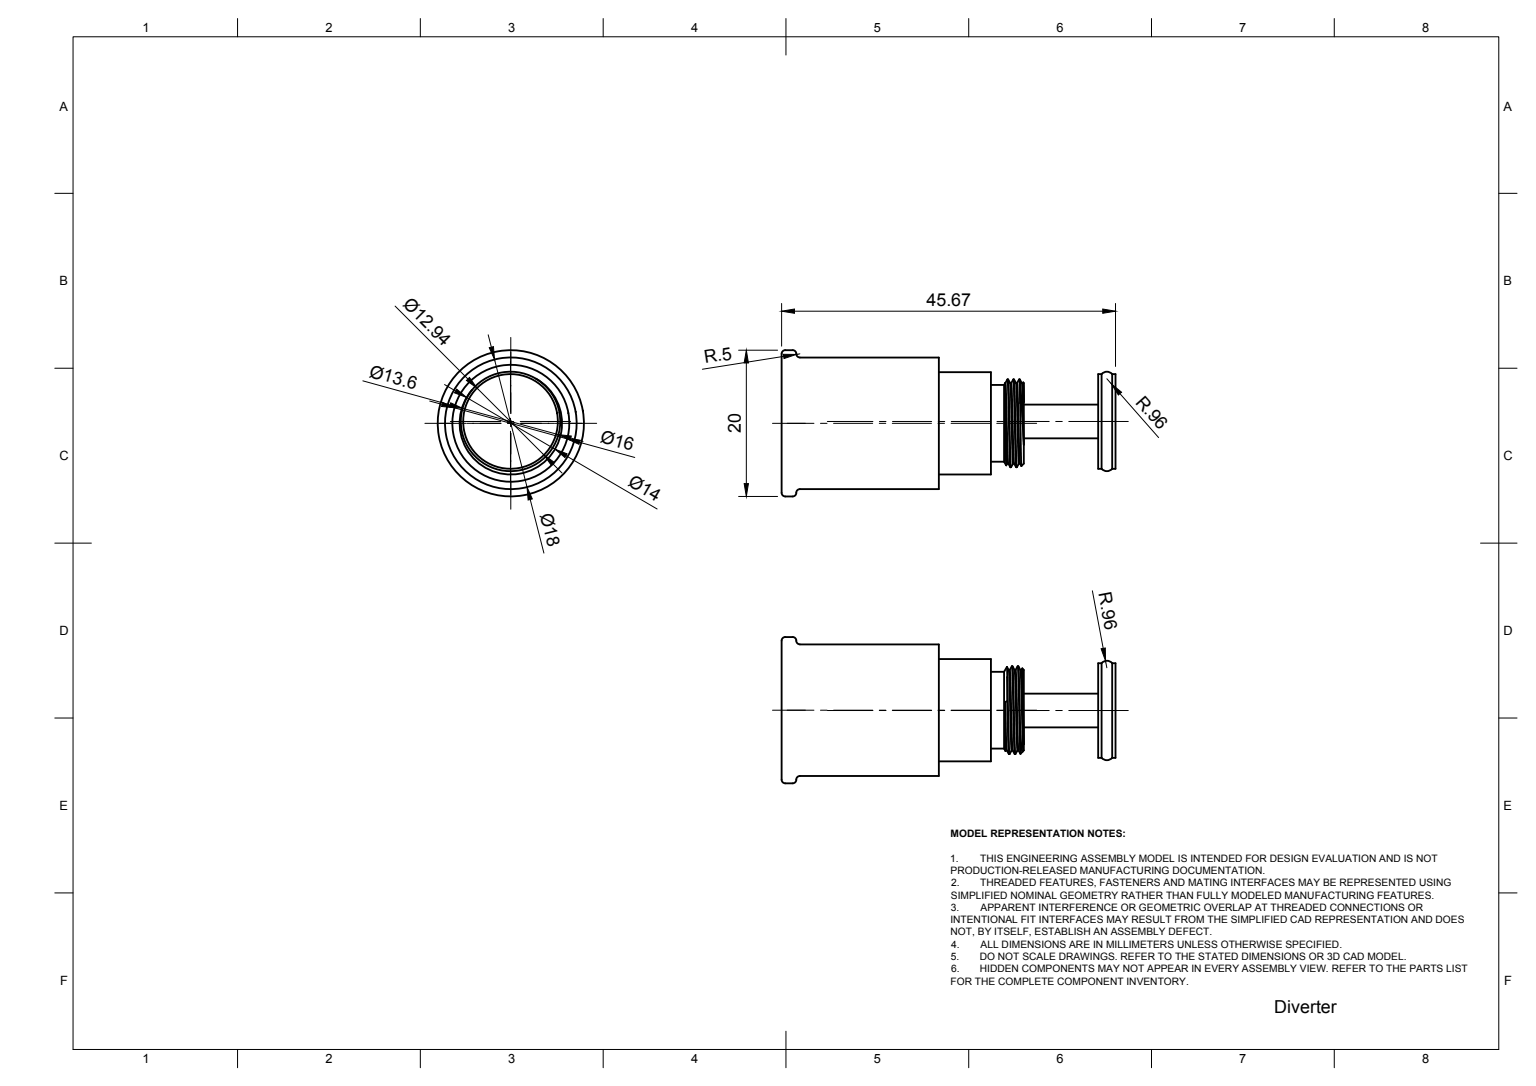
ISO-10303-21;
HEADER;
/* Generated by software containing ST-Developer
 * from STEP Tools, Inc. (www.steptools.com) 
 */

FILE_DESCRIPTION(
/* description */ ('STEP AP214'),
/* implementation_level */ '2;1');

FILE_NAME(
/* name */ 'Diverter.step',
/* time_stamp */ '2026-10-05T23:18:41-07:00',
/* author */ (''),
/* organization */ (''),
/* preprocessor_version */ 'ST-DEVELOPER v20.2',
/* originating_system */ 'Autodesk Translation Framework v15.15.0.0',
/* authorisation */ '');

FILE_SCHEMA (('AUTOMOTIVE_DESIGN { 1 0 10303 214 3 1 1 }'));
ENDSEC;

DATA;
#10=MECHANICAL_DESIGN_GEOMETRIC_PRESENTATION_REPRESENTATION('',(#108),#221662);
#82=SHAPE_REPRESENTATION_RELATIONSHIP('SRR','None',#221717,#95);
#95=ADVANCED_BREP_SHAPE_REPRESENTATION('',(#79337),#221657);
#108=STYLED_ITEM('',(#221783),#79337);
#199=B_SPLINE_SURFACE_WITH_KNOTS('',1,3,((#183512,#183513,#183514,#183515,
#183516,#183517,#183518,#183519,#183520,#183521,#183522,#183523,#183524,
#183525,#183526,#183527,#183528,#183529,#183530,#183531,#183532,#183533,
#183534,#183535,#183536,#183537,#183538,#183539,#183540,#183541,#183542,
#183543,#183544,#183545,#183546,#183547,#183548,#183549,#183550,#183551,
#183552,#183553,#183554,#183555,#183556,#183557,#183558,#183559,#183560,
#183561,#183562,#183563,#183564,#183565),(#183566,#183567,#183568,#183569,
#183570,#183571,#183572,#183573,#183574,#183575,#183576,#183577,#183578,
#183579,#183580,#183581,#183582,#183583,#183584,#183585,#183586,#183587,
#183588,#183589,#183590,#183591,#183592,#183593,#183594,#183595,#183596,
#183597,#183598,#183599,#183600,#183601,#183602,#183603,#183604,#183605,
#183606,#183607,#183608,#183609,#183610,#183611,#183612,#183613,#183614,
#183615,#183616,#183617,#183618,#183619)),.UNSPECIFIED.,.F.,.F.,.F.,(2,
2),(4,1,1,1,1,1,1,1,1,1,1,1,1,1,1,1,1,1,1,1,1,1,1,1,1,1,1,1,1,1,1,1,1,1,
1,1,1,1,1,1,1,1,1,1,1,1,1,1,1,1,1,4),(0.,1.),(0.,0.0198373427721521,0.0396746855443041,
0.0595120283164562,0.0793493710886083,0.0991867138607603,0.119024056632912,
0.138861399405064,0.158698742177217,0.178536084949369,0.198373427721521,
0.218210770493673,0.238048113265825,0.257885456037977,0.277722798810129,
0.297560141582281,0.317397484354433,0.337234827126585,0.357072169898737,
0.376909512670889,0.396746855443041,0.416584198215193,0.436421540987345,
0.456258883759498,0.47609622653165,0.495933569303802,0.515770912075954,
0.535608254848106,0.555445597620258,0.57528294039241,0.595120283164562,
0.614957625936714,0.634794968708866,0.654632311481018,0.67446965425317,
0.694306997025322,0.714144339797474,0.733981682569626,0.753819025341778,
0.773656368113931,0.793493710886083,0.813331053658235,0.833168396430387,
0.853005739202539,0.872843081974691,0.892680424746843,0.912517767518995,
0.932355110291147,0.952192453063299,0.972029795835451,0.991867138607603,
1.),.UNSPECIFIED.);
#200=B_SPLINE_SURFACE_WITH_KNOTS('',1,3,((#183620,#183621,#183622,#183623,
#183624,#183625,#183626,#183627,#183628,#183629,#183630,#183631,#183632,
#183633,#183634,#183635,#183636,#183637,#183638,#183639,#183640,#183641,
#183642,#183643,#183644,#183645,#183646,#183647,#183648,#183649,#183650,
#183651,#183652,#183653,#183654,#183655,#183656,#183657,#183658,#183659,
#183660,#183661,#183662,#183663,#183664,#183665,#183666,#183667,#183668,
#183669,#183670,#183671,#183672,#183673),(#183674,#183675,#183676,#183677,
#183678,#183679,#183680,#183681,#183682,#183683,#183684,#183685,#183686,
#183687,#183688,#183689,#183690,#183691,#183692,#183693,#183694,#183695,
#183696,#183697,#183698,#183699,#183700,#183701,#183702,#183703,#183704,
#183705,#183706,#183707,#183708,#183709,#183710,#183711,#183712,#183713,
#183714,#183715,#183716,#183717,#183718,#183719,#183720,#183721,#183722,
#183723,#183724,#183725,#183726,#183727)),.UNSPECIFIED.,.F.,.F.,.F.,(2,
2),(4,1,1,1,1,1,1,1,1,1,1,1,1,1,1,1,1,1,1,1,1,1,1,1,1,1,1,1,1,1,1,1,1,1,
1,1,1,1,1,1,1,1,1,1,1,1,1,1,1,1,1,4),(0.,1.),(0.,0.0198373427721521,0.0396746855443041,
0.0595120283164562,0.0793493710886083,0.0991867138607603,0.119024056632912,
0.138861399405064,0.158698742177217,0.178536084949369,0.198373427721521,
0.218210770493673,0.238048113265825,0.257885456037977,0.277722798810129,
0.297560141582281,0.317397484354433,0.337234827126585,0.357072169898737,
0.376909512670889,0.396746855443041,0.416584198215193,0.436421540987345,
0.456258883759498,0.47609622653165,0.495933569303802,0.515770912075954,
0.535608254848106,0.555445597620258,0.57528294039241,0.595120283164562,
0.614957625936714,0.634794968708866,0.654632311481018,0.67446965425317,
0.694306997025322,0.714144339797474,0.733981682569626,0.753819025341778,
0.773656368113931,0.793493710886083,0.813331053658235,0.833168396430387,
0.853005739202539,0.872843081974691,0.892680424746843,0.912517767518995,
0.932355110291147,0.952192453063299,0.972029795835451,0.991867138607603,
1.),.UNSPECIFIED.);
#305=FACE_BOUND('',#24899,.T.);
#306=FACE_BOUND('',#24901,.T.);
#307=FACE_BOUND('',#24903,.T.);
#308=FACE_BOUND('',#24906,.T.);
#309=FACE_BOUND('',#24909,.T.);
#310=FACE_BOUND('',#24917,.T.);
#311=FACE_BOUND('',#24919,.T.);
#312=FACE_BOUND('',#24921,.T.);
#313=FACE_BOUND('',#24924,.T.);
#1800=(
BOUNDED_CURVE()
B_SPLINE_CURVE(2,(#182624,#182625,#182626),.UNSPECIFIED.,.F.,.F.)
B_SPLINE_CURVE_WITH_KNOTS((3,3),(0.462569328702153,0.587652141350747),
 .UNSPECIFIED.)
CURVE()
GEOMETRIC_REPRESENTATION_ITEM()
RATIONAL_B_SPLINE_CURVE((1.3055338176145,1.33529904244958,1.35882091219323))
REPRESENTATION_ITEM('')
);
#1801=(
BOUNDED_CURVE()
B_SPLINE_CURVE(2,(#183748,#183749,#183750),.UNSPECIFIED.,.F.,.F.)
B_SPLINE_CURVE_WITH_KNOTS((3,3),(-1.97427612804245,-1.83367684633348),
 .UNSPECIFIED.)
CURVE()
GEOMETRIC_REPRESENTATION_ITEM()
RATIONAL_B_SPLINE_CURVE((1.43398246254344,1.46667622338746,1.49251235895387))
REPRESENTATION_ITEM('')
);
#1898=TOROIDAL_SURFACE('',#80902,5.84208667428926,0.959420631745662);
#1899=TOROIDAL_SURFACE('',#80915,9.5,0.5);
#1900=TOROIDAL_SURFACE('',#80918,9.5,0.5);
#1901=TOROIDAL_SURFACE('',#80921,9.5,0.5);
#1902=TOROIDAL_SURFACE('',#80926,7.5,0.5);
#1947=CONICAL_SURFACE('',#80853,2.05,1.0297442575);
#1948=CONICAL_SURFACE('',#80859,5.5,0.7853981625);
#1949=CONICAL_SURFACE('',#80871,7.,0.7853981625);
#1950=CONICAL_SURFACE('',#80878,6.,1.04719755);
#1951=CONICAL_SURFACE('',#80890,2.55,0.7853981625);
#1952=CONICAL_SURFACE('',#80892,3.05,0.7853981625);
#1953=CONICAL_SURFACE('',#80894,5.5,0.7853981625);
#1954=CONICAL_SURFACE('',#80896,4.9,0.7853981625);
#1955=CONICAL_SURFACE('',#80948,7.,0.7853981625);
#1979=ORIENTED_CLOSED_SHELL('',*,#79330,.F.);
#2254=CYLINDRICAL_SURFACE('',#80849,2.05);
#2255=CYLINDRICAL_SURFACE('',#80855,5.5);
#2256=CYLINDRICAL_SURFACE('',#80857,5.5);
#2257=CYLINDRICAL_SURFACE('',#80858,5.5);
#2258=CYLINDRICAL_SURFACE('',#80861,6.);
#2259=CYLINDRICAL_SURFACE('',#80863,6.);
#2260=CYLINDRICAL_SURFACE('',#80864,7.);
#2261=CYLINDRICAL_SURFACE('',#80873,5.25);
#2262=CYLINDRICAL_SURFACE('',#80876,6.);
#2263=CYLINDRICAL_SURFACE('',#80881,4.4);
#2264=CYLINDRICAL_SURFACE('',#80885,2.55);
#2265=CYLINDRICAL_SURFACE('',#80898,5.5);
#2266=CYLINDRICAL_SURFACE('',#80899,6.47238979616114);
#2267=CYLINDRICAL_SURFACE('',#80905,6.47238979616113);
#2268=CYLINDRICAL_SURFACE('',#80907,9.);
#2269=CYLINDRICAL_SURFACE('',#80911,9.99999999999999);
#2270=CYLINDRICAL_SURFACE('',#80923,7.99999999999999);
#2271=CYLINDRICAL_SURFACE('',#80929,4.);
#2272=CYLINDRICAL_SURFACE('',#80932,2.30850939467147);
#3188=LINE('',#181115,#10255);
#3189=LINE('',#181121,#10256);
#3190=LINE('',#181126,#10257);
#3191=LINE('',#181319,#10258);
#3192=LINE('',#181683,#10259);
#3193=LINE('',#182045,#10260);
#3194=LINE('',#182068,#10261);
#3195=LINE('',#182209,#10262);
#3196=LINE('',#182592,#10263);
#3197=LINE('',#182596,#10264);
#3198=LINE('',#182600,#10265);
#3199=LINE('',#182604,#10266);
#3200=LINE('',#182608,#10267);
#3201=LINE('',#182631,#10268);
#3202=LINE('',#183011,#10269);
#3203=LINE('',#183017,#10270);
#3204=LINE('',#183027,#10271);
#3205=LINE('',#183032,#10272);
#3206=LINE('',#183043,#10273);
#3207=LINE('',#183054,#10274);
#3208=LINE('',#183187,#10275);
#3209=LINE('',#183448,#10276);
#3210=LINE('',#183456,#10277);
#3211=LINE('',#183463,#10278);
#3212=LINE('',#183470,#10279);
#3213=LINE('',#183488,#10280);
#3214=LINE('',#183498,#10281);
#3215=LINE('',#183504,#10282);
#3216=LINE('',#183729,#10283);
#3217=LINE('',#183742,#10284);
#3218=LINE('',#183744,#10285);
#3219=LINE('',#183747,#10286);
#10255=VECTOR('',#89389,2.05);
#10256=VECTOR('',#89396,2.05);
#10257=VECTOR('',#89401,5.5);
#10258=VECTOR('',#89406,5.5);
#10259=VECTOR('',#89409,5.5);
#10260=VECTOR('',#89412,5.5);
#10261=VECTOR('',#89417,6.);
#10262=VECTOR('',#89422,6.);
#10263=VECTOR('',#89427,7.);
#10264=VECTOR('',#89430,1000.);
#10265=VECTOR('',#89433,1000.);
#10266=VECTOR('',#89436,1000.);
#10267=VECTOR('',#89439,1000.);
#10268=VECTOR('',#89450,5.25);
#10269=VECTOR('',#89463,6.);
#10270=VECTOR('',#89468,4.4);
#10271=VECTOR('',#89479,1000.);
#10272=VECTOR('',#89484,1000.);
#10273=VECTOR('',#89487,2.55);
#10274=VECTOR('',#89492,3.05);
#10275=VECTOR('',#89501,4.9);
#10276=VECTOR('',#89510,6.47238979616114);
#10277=VECTOR('',#89521,6.47238979616113);
#10278=VECTOR('',#89528,9.);
#10279=VECTOR('',#89537,9.99999999999999);
#10280=VECTOR('',#89562,8.);
#10281=VECTOR('',#89575,4.);
#10282=VECTOR('',#89582,2.30850939467147);
#10283=VECTOR('',#89599,1000.);
#10284=VECTOR('',#89602,1000.);
#10285=VECTOR('',#89605,1000.);
#10286=VECTOR('',#89608,1000.);
#17003=PLANE('',#80854);
#17004=PLANE('',#80935);
#17005=PLANE('',#80936);
#17006=PLANE('',#80937);
#17007=PLANE('',#80938);
#17008=PLANE('',#80939);
#17009=PLANE('',#80940);
#17010=PLANE('',#80941);
#17011=PLANE('',#80942);
#17012=PLANE('',#80943);
#17013=PLANE('',#80944);
#17014=PLANE('',#80945);
#17015=PLANE('',#80946);
#17016=PLANE('',#80947);
#17017=PLANE('',#80950);
#20791=FACE_OUTER_BOUND('',#24866,.T.);
#20792=FACE_OUTER_BOUND('',#24867,.T.);
#20793=FACE_OUTER_BOUND('',#24868,.T.);
#20794=FACE_OUTER_BOUND('',#24869,.T.);
#20795=FACE_OUTER_BOUND('',#24870,.T.);
#20796=FACE_OUTER_BOUND('',#24871,.T.);
#20797=FACE_OUTER_BOUND('',#24872,.T.);
#20798=FACE_OUTER_BOUND('',#24873,.T.);
#20799=FACE_OUTER_BOUND('',#24874,.T.);
#20800=FACE_OUTER_BOUND('',#24875,.T.);
#20801=FACE_OUTER_BOUND('',#24876,.T.);
#20802=FACE_OUTER_BOUND('',#24877,.T.);
#20803=FACE_OUTER_BOUND('',#24878,.T.);
#20804=FACE_OUTER_BOUND('',#24879,.T.);
#20805=FACE_OUTER_BOUND('',#24880,.T.);
#20806=FACE_OUTER_BOUND('',#24881,.T.);
#20807=FACE_OUTER_BOUND('',#24882,.T.);
#20808=FACE_OUTER_BOUND('',#24883,.T.);
#20809=FACE_OUTER_BOUND('',#24884,.T.);
#20810=FACE_OUTER_BOUND('',#24885,.T.);
#20811=FACE_OUTER_BOUND('',#24886,.T.);
#20812=FACE_OUTER_BOUND('',#24887,.T.);
#20813=FACE_OUTER_BOUND('',#24888,.T.);
#20814=FACE_OUTER_BOUND('',#24889,.T.);
#20815=FACE_OUTER_BOUND('',#24890,.T.);
#20816=FACE_OUTER_BOUND('',#24891,.T.);
#20817=FACE_OUTER_BOUND('',#24892,.T.);
#20818=FACE_OUTER_BOUND('',#24893,.T.);
#20819=FACE_OUTER_BOUND('',#24894,.T.);
#20820=FACE_OUTER_BOUND('',#24895,.T.);
#20821=FACE_OUTER_BOUND('',#24896,.T.);
#20822=FACE_OUTER_BOUND('',#24897,.T.);
#20823=FACE_OUTER_BOUND('',#24898,.T.);
#20824=FACE_OUTER_BOUND('',#24900,.T.);
#20825=FACE_OUTER_BOUND('',#24902,.T.);
#20826=FACE_OUTER_BOUND('',#24904,.T.);
#20827=FACE_OUTER_BOUND('',#24905,.T.);
#20828=FACE_OUTER_BOUND('',#24907,.T.);
#20829=FACE_OUTER_BOUND('',#24908,.T.);
#20830=FACE_OUTER_BOUND('',#24910,.T.);
#20831=FACE_OUTER_BOUND('',#24911,.T.);
#20832=FACE_OUTER_BOUND('',#24912,.T.);
#20833=FACE_OUTER_BOUND('',#24913,.T.);
#20834=FACE_OUTER_BOUND('',#24914,.T.);
#20835=FACE_OUTER_BOUND('',#24915,.T.);
#20836=FACE_OUTER_BOUND('',#24916,.T.);
#20837=FACE_OUTER_BOUND('',#24918,.T.);
#20838=FACE_OUTER_BOUND('',#24920,.T.);
#20839=FACE_OUTER_BOUND('',#24922,.T.);
#20840=FACE_OUTER_BOUND('',#24923,.T.);
#24866=EDGE_LOOP('',(#56903,#56904,#56905,#56906,#56907));
#24867=EDGE_LOOP('',(#56908,#56909,#56910,#56911));
#24868=EDGE_LOOP('',(#56912));
#24869=EDGE_LOOP('',(#56913,#56914,#56915,#56916));
#24870=EDGE_LOOP('',(#56917,#56918,#56919,#56920));
#24871=EDGE_LOOP('',(#56921,#56922,#56923,#56924));
#24872=EDGE_LOOP('',(#56925,#56926,#56927));
#24873=EDGE_LOOP('',(#56928,#56929,#56930,#56931));
#24874=EDGE_LOOP('',(#56932,#56933,#56934,#56935));
#24875=EDGE_LOOP('',(#56936,#56937,#56938,#56939,#56940,#56941,#56942,#56943,
#56944,#56945,#56946,#56947));
#24876=EDGE_LOOP('',(#56948,#56949,#56950,#56951));
#24877=EDGE_LOOP('',(#56952,#56953,#56954,#56955));
#24878=EDGE_LOOP('',(#56956,#56957,#56958,#56959));
#24879=EDGE_LOOP('',(#56960,#56961,#56962,#56963,#56964,#56965,#56966,#56967));
#24880=EDGE_LOOP('',(#56968,#56969,#56970,#56971,#56972));
#24881=EDGE_LOOP('',(#56973,#56974,#56975,#56976,#56977,#56978));
#24882=EDGE_LOOP('',(#56979,#56980,#56981,#56982,#56983,#56984));
#24883=EDGE_LOOP('',(#56985,#56986,#56987,#56988,#56989,#56990));
#24884=EDGE_LOOP('',(#56991,#56992,#56993,#56994,#56995,#56996));
#24885=EDGE_LOOP('',(#56997,#56998,#56999,#57000,#57001));
#24886=EDGE_LOOP('',(#57002,#57003,#57004,#57005));
#24887=EDGE_LOOP('',(#57006,#57007,#57008,#57009));
#24888=EDGE_LOOP('',(#57010,#57011,#57012,#57013));
#24889=EDGE_LOOP('',(#57014,#57015,#57016,#57017));
#24890=EDGE_LOOP('',(#57018,#57019,#57020,#57021,#57022));
#24891=EDGE_LOOP('',(#57023,#57024,#57025,#57026,#57027));
#24892=EDGE_LOOP('',(#57028,#57029,#57030,#57031));
#24893=EDGE_LOOP('',(#57032,#57033,#57034,#57035,#57036));
#24894=EDGE_LOOP('',(#57037,#57038,#57039,#57040,#57041));
#24895=EDGE_LOOP('',(#57042,#57043,#57044,#57045));
#24896=EDGE_LOOP('',(#57046,#57047,#57048,#57049));
#24897=EDGE_LOOP('',(#57050,#57051,#57052,#57053));
#24898=EDGE_LOOP('',(#57054,#57055,#57056,#57057));
#24899=EDGE_LOOP('',(#57058,#57059,#57060,#57061));
#24900=EDGE_LOOP('',(#57062));
#24901=EDGE_LOOP('',(#57063));
#24902=EDGE_LOOP('',(#57064));
#24903=EDGE_LOOP('',(#57065));
#24904=EDGE_LOOP('',(#57066));
#24905=EDGE_LOOP('',(#57067));
#24906=EDGE_LOOP('',(#57068));
#24907=EDGE_LOOP('',(#57069));
#24908=EDGE_LOOP('',(#57070));
#24909=EDGE_LOOP('',(#57071));
#24910=EDGE_LOOP('',(#57072,#57073,#57074,#57075,#57076,#57077,#57078,#57079,
#57080,#57081,#57082));
#24911=EDGE_LOOP('',(#57083,#57084,#57085,#57086,#57087,#57088,#57089,#57090,
#57091,#57092));
#24912=EDGE_LOOP('',(#57093,#57094));
#24913=EDGE_LOOP('',(#57095,#57096,#57097,#57098,#57099,#57100));
#24914=EDGE_LOOP('',(#57101,#57102));
#24915=EDGE_LOOP('',(#57103,#57104,#57105,#57106,#57107,#57108));
#24916=EDGE_LOOP('',(#57109));
#24917=EDGE_LOOP('',(#57110));
#24918=EDGE_LOOP('',(#57111,#57112,#57113));
#24919=EDGE_LOOP('',(#57114));
#24920=EDGE_LOOP('',(#57115));
#24921=EDGE_LOOP('',(#57116));
#24922=EDGE_LOOP('',(#57117,#57118,#57119,#57120,#57121));
#24923=EDGE_LOOP('',(#57122,#57123,#57124,#57125));
#24924=EDGE_LOOP('',(#57126));
#30274=B_SPLINE_CURVE_WITH_KNOTS('',3,(#181128,#181129,#181130,#181131,
#181132,#181133,#181134,#181135,#181136,#181137,#181138,#181139,#181140,
#181141,#181142,#181143,#181144,#181145,#181146,#181147,#181148,#181149,
#181150,#181151,#181152,#181153,#181154,#181155,#181156,#181157,#181158,
#181159,#181160,#181161,#181162,#181163,#181164,#181165,#181166,#181167,
#181168,#181169,#181170,#181171,#181172,#181173,#181174,#181175,#181176,
#181177,#181178,#181179,#181180,#181181,#181182,#181183,#181184,#181185,
#181186,#181187,#181188,#181189,#181190,#181191,#181192,#181193,#181194,
#181195,#181196,#181197,#181198,#181199,#181200,#181201,#181202,#181203,
#181204,#181205,#181206,#181207,#181208,#181209,#181210,#181211,#181212,
#181213,#181214,#181215,#181216,#181217,#181218,#181219,#181220,#181221,
#181222,#181223,#181224,#181225,#181226,#181227,#181228,#181229,#181230,
#181231,#181232,#181233,#181234,#181235,#181236,#181237),.UNSPECIFIED.,
 .F.,.F.,(4,2,2,2,2,2,2,2,2,2,2,2,2,2,2,2,2,2,2,2,2,2,2,2,2,2,2,2,2,2,2,
2,2,2,2,2,2,2,2,2,2,2,2,2,2,2,2,2,2,2,2,2,2,2,4),(-2.0374264169892,-2.03325723873566,
-2.01852518698755,-1.98019546730744,-1.89910957670444,-1.8473559268582,
-1.82181501438801,-1.8000221301294,-1.77132035516003,-1.73779453405823,
-1.65621553961038,-1.62324600384763,-1.60802171249166,-1.59508722455329,
-1.57328737753901,-1.54369621600048,-1.43275430172482,-1.40641781973598,
-1.3848882552916,-1.35742036745476,-1.2746876774316,-1.19931109475228,-1.18126032660081,
-1.16953462805175,-1.15525014334195,-1.12077741049727,-1.05645337488967,
-0.986844591638145,-0.96000395932419,-0.938279265882365,-0.911240690812327,
-0.880604952539318,-0.816126256851267,-0.76177602608691,-0.745553142489823,
-0.733025997958031,-0.713891980393471,-0.689464491039709,-0.623696595424254,
-0.566646952663267,-0.540885267446727,-0.519111084586999,-0.490775715375377,
-0.413973876129471,-0.333776908151955,-0.316301768502787,-0.304639059444405,
-0.290026744158241,-0.252788348082332,-0.176955717799064,-0.119916186580509,
-0.093942455038947,-0.0721880153941974,-0.0510648498280456,-0.000149360373092413),
 .UNSPECIFIED.);
#30275=B_SPLINE_CURVE_WITH_KNOTS('',3,(#181240,#181241,#181242,#181243,
#181244,#181245,#181246,#181247,#181248,#181249,#181250,#181251,#181252,
#181253,#181254,#181255,#181256,#181257,#181258,#181259,#181260,#181261,
#181262,#181263,#181264,#181265,#181266,#181267,#181268,#181269,#181270,
#181271,#181272,#181273,#181274,#181275,#181276,#181277,#181278,#181279,
#181280,#181281,#181282,#181283,#181284,#181285,#181286,#181287,#181288,
#181289,#181290,#181291,#181292,#181293,#181294,#181295,#181296,#181297,
#181298,#181299,#181300,#181301,#181302,#181303,#181304,#181305,#181306,
#181307,#181308,#181309,#181310,#181311,#181312,#181313,#181314,#181315),
 .UNSPECIFIED.,.F.,.F.,(4,2,2,2,2,2,2,2,2,2,2,2,2,2,2,2,2,2,2,2,2,2,2,2,
2,2,2,2,2,2,2,2,2,2,2,2,2,4),(-11.0420177746592,-10.9599397421387,-10.9398938962619,
-10.923237123713,-10.9106052415203,-10.8947670479531,-10.8078828554248,
-10.7438996772105,-10.718208157378,-10.6964285618455,-10.6684886275246,
-10.5730160503389,-10.5086930824629,-10.4924060260972,-10.4808258283884,
-10.4656213586583,-10.4259108932372,-10.3590662985945,-10.2972473633837,
-10.2713228294197,-10.2495656322461,-10.2219108414823,-10.1537182957188,
-10.1005077442629,-10.0783068470237,-10.0604069299075,-10.0478241035653,
-10.0302281109333,-9.95833483875728,-9.88365573874688,-9.85656659541233,
-9.83484229672353,-9.80805159221074,-9.741502251406,-9.67479042103899,-9.63969737588758,
-9.6253365275997,-9.62176322384599),.UNSPECIFIED.);
#30276=B_SPLINE_CURVE_WITH_KNOTS('',3,(#181320,#181321,#181322,#181323,
#181324,#181325,#181326,#181327,#181328,#181329,#181330,#181331,#181332,
#181333,#181334,#181335,#181336,#181337,#181338,#181339,#181340,#181341,
#181342,#181343,#181344,#181345,#181346,#181347,#181348,#181349,#181350,
#181351,#181352,#181353,#181354,#181355,#181356,#181357,#181358,#181359,
#181360,#181361,#181362,#181363,#181364,#181365,#181366,#181367,#181368,
#181369,#181370,#181371,#181372,#181373,#181374,#181375,#181376,#181377,
#181378,#181379,#181380,#181381,#181382,#181383,#181384,#181385,#181386,
#181387,#181388,#181389,#181390,#181391,#181392,#181393,#181394,#181395,
#181396,#181397,#181398,#181399,#181400,#181401,#181402,#181403,#181404,
#181405,#181406,#181407,#181408,#181409,#181410,#181411,#181412,#181413,
#181414,#181415,#181416,#181417,#181418,#181419,#181420,#181421,#181422,
#181423,#181424,#181425,#181426,#181427,#181428,#181429,#181430,#181431,
#181432,#181433,#181434,#181435,#181436,#181437,#181438,#181439,#181440,
#181441,#181442,#181443,#181444,#181445,#181446,#181447,#181448,#181449,
#181450,#181451,#181452,#181453,#181454,#181455,#181456,#181457,#181458,
#181459,#181460,#181461,#181462,#181463,#181464,#181465,#181466,#181467,
#181468,#181469,#181470,#181471,#181472,#181473,#181474,#181475,#181476,
#181477,#181478,#181479,#181480,#181481,#181482,#181483,#181484,#181485,
#181486,#181487,#181488,#181489,#181490,#181491,#181492,#181493,#181494,
#181495,#181496,#181497,#181498,#181499,#181500,#181501),.UNSPECIFIED.,
 .F.,.F.,(4,2,2,2,2,2,2,2,2,2,2,2,2,2,2,2,2,2,2,2,2,2,2,2,2,2,2,2,2,2,2,
2,2,2,2,2,2,2,2,2,2,2,2,2,2,2,2,2,2,2,2,2,2,2,2,2,2,2,2,2,2,2,2,2,2,2,2,
2,2,2,2,2,2,2,2,2,2,2,2,2,2,2,2,2,2,2,2,2,2,2,4),(-5.49514095832648,-5.49479992473117,
-5.4820584180547,-5.45783766717952,-5.32910650724132,-5.29327873109851,
-5.27057092541286,-5.24752547378678,-5.20900193213987,-5.15508416570214,
-5.08711236100685,-5.06926421126503,-5.05668133832967,-5.03903409214227,
-4.97994615985857,-4.89316178777948,-4.86585298026823,-4.84412509360188,
-4.8175347032467,-4.74555196018678,-4.6567371781831,-4.63879628292061,-4.62708350973762,
-4.61274018657622,-4.57779243715063,-4.51164856045253,-4.44461999984613,
-4.41773445466564,-4.39600985688239,-4.36901756354521,-4.29343048511146,
-4.22225763360175,-4.20461264184201,-4.19202980445917,-4.1741794951694,
-4.15206701369583,-4.09929898265307,-4.03042520549459,-4.00278967559688,
-3.98103278125623,-3.95509190484458,-3.89308759144006,-3.82620275634084,
-3.78665450219168,-3.77148423019889,-3.7599021211164,-3.74357271272327,
-3.6768433017597,-3.58444871147446,-3.55629077886608,-3.53449449496795,
-3.50895308800941,-3.44738813407108,-3.37754034248968,-3.34859811288362,
-3.33456473684734,-3.32095844719234,-3.29475388264289,-3.25528548292294,
-3.16310634592479,-3.1362527942936,-3.1145276481891,-3.08750362661562,-3.05726646565273,
-2.9971538208965,-2.92816109205382,-2.91012982645738,-2.89840655169761,
-2.88411199446826,-2.84955770748755,-2.78492463024832,-2.71575655695739,
-2.68890888665255,-2.66718444560362,-2.64015373933234,-2.62408225637449,
-2.6010943112649,-2.51599344191209,-2.48792465828078,-2.47261609198703,
-2.45971084992899,-2.43812581613357,-2.4089703937702,-2.30143419560341,
-2.2738713464661,-2.25211855318578,-2.22612269040889,-2.16343062428365,
-2.0621869162582,-2.04490192589283,-2.0374264169892),.UNSPECIFIED.);
#30277=B_SPLINE_CURVE_WITH_KNOTS('',3,(#181502,#181503,#181504,#181505,
#181506,#181507,#181508,#181509,#181510,#181511,#181512,#181513,#181514,
#181515,#181516,#181517,#181518,#181519,#181520,#181521,#181522,#181523,
#181524,#181525,#181526,#181527,#181528,#181529,#181530,#181531,#181532,
#181533,#181534,#181535,#181536,#181537,#181538,#181539,#181540,#181541,
#181542,#181543,#181544,#181545,#181546,#181547,#181548,#181549,#181550,
#181551,#181552,#181553,#181554,#181555,#181556,#181557,#181558,#181559,
#181560,#181561,#181562,#181563,#181564,#181565,#181566,#181567,#181568,
#181569,#181570,#181571,#181572,#181573,#181574,#181575,#181576,#181577,
#181578,#181579,#181580,#181581,#181582,#181583,#181584,#181585,#181586,
#181587,#181588,#181589,#181590,#181591,#181592,#181593,#181594,#181595,
#181596,#181597,#181598,#181599,#181600,#181601,#181602,#181603,#181604,
#181605,#181606,#181607,#181608,#181609,#181610,#181611,#181612,#181613,
#181614,#181615,#181616,#181617,#181618,#181619,#181620,#181621,#181622,
#181623,#181624,#181625,#181626,#181627,#181628,#181629,#181630,#181631,
#181632,#181633,#181634,#181635,#181636,#181637,#181638,#181639,#181640,
#181641,#181642,#181643,#181644,#181645,#181646,#181647,#181648,#181649,
#181650,#181651,#181652,#181653,#181654,#181655,#181656,#181657,#181658,
#181659,#181660,#181661,#181662,#181663,#181664,#181665,#181666,#181667,
#181668,#181669,#181670,#181671,#181672,#181673,#181674,#181675,#181676,
#181677,#181678,#181679),.UNSPECIFIED.,.F.,.F.,(4,2,2,2,2,2,2,2,2,2,2,2,
2,2,2,2,2,2,2,2,2,2,2,2,2,2,2,2,2,2,2,2,2,2,2,2,2,2,2,2,2,2,2,2,2,2,2,2,
2,2,2,2,2,2,2,2,2,2,2,2,2,2,2,2,2,2,2,2,2,2,2,2,2,2,2,2,2,2,2,2,2,2,2,2,
2,2,2,2,4),(-9.62176322384599,-9.61362793664136,-9.59572068391397,-9.51842556037379,
-9.43864125932449,-9.41068969274724,-9.3889379954071,-9.36289536573885,
-9.29603888750942,-9.21996859001137,-9.1990239946575,-9.18620176302793,
-9.17061958148039,-9.13357698038007,-9.0557120872312,-9.02273687179219,
-8.9943474525171,-8.97257599227928,-8.94683145156729,-8.89339699252227,
-8.81415845666444,-8.77620113787093,-8.76150967376524,-8.74985971603038,
-8.73251307255491,-8.6388488468192,-8.57001675505747,-8.54359818107113,
-8.52186669522419,-8.49436302458913,-8.41214561447724,-8.36754232123613,
-8.34719712953825,-8.33036481139516,-8.3177486818033,-8.30208368864063,
-8.2570642930598,-8.18778763062589,-8.15624359064142,-8.12867597788388,
-8.10694230403665,-8.08057669381003,-8.01636404010515,-7.94695688957519,
-7.91119382815484,-7.89675209882627,-7.88505957115733,-7.86729663388556,
-7.77608614635548,-7.7058864190148,-7.67938958125659,-7.65765989890923,
-7.63024603986514,-7.54551338030752,-7.48324689940725,-7.46622800531952,
-7.45362464997324,-7.43813235833985,-7.35698949434093,-7.29194643889332,
-7.2643374505598,-7.24260214694485,-7.21627009228013,-7.15987645830453,
-7.0843738374995,-7.04720640187818,-7.03260202344148,-7.02093811517747,
-7.00345032242073,-6.91062255393296,-6.84132138876095,-6.81487464097661,
-6.79314319744251,-6.76567040428183,-6.6824952859288,-6.62038536131578,
-6.60266652125036,-6.59008399296299,-6.57230887829423,-6.50314991168874,
-6.44984717547513,-6.41157111664384,-6.38856109819059,-6.36582284170627,
-6.32979323434818,-6.22610083519746,-6.1840247938677,-6.16892022716619,
-6.16419090700929),.UNSPECIFIED.);
#30278=B_SPLINE_CURVE_WITH_KNOTS('',3,(#181684,#181685,#181686,#181687,
#181688,#181689,#181690,#181691,#181692,#181693,#181694,#181695,#181696,
#181697,#181698,#181699,#181700,#181701,#181702,#181703,#181704,#181705,
#181706,#181707,#181708,#181709,#181710,#181711,#181712,#181713,#181714,
#181715,#181716,#181717,#181718,#181719,#181720,#181721,#181722,#181723,
#181724,#181725,#181726,#181727,#181728,#181729,#181730,#181731,#181732,
#181733,#181734,#181735,#181736,#181737,#181738,#181739,#181740,#181741,
#181742,#181743,#181744,#181745,#181746,#181747,#181748,#181749,#181750,
#181751,#181752,#181753,#181754,#181755,#181756,#181757,#181758,#181759,
#181760,#181761,#181762,#181763,#181764,#181765,#181766,#181767,#181768,
#181769,#181770,#181771,#181772,#181773,#181774,#181775,#181776,#181777,
#181778,#181779,#181780,#181781,#181782,#181783,#181784,#181785,#181786,
#181787,#181788,#181789,#181790,#181791,#181792,#181793,#181794,#181795,
#181796,#181797,#181798,#181799,#181800,#181801,#181802,#181803,#181804,
#181805,#181806,#181807,#181808,#181809,#181810,#181811,#181812,#181813,
#181814,#181815,#181816,#181817,#181818,#181819,#181820,#181821,#181822,
#181823,#181824,#181825,#181826,#181827,#181828,#181829,#181830,#181831,
#181832,#181833,#181834,#181835,#181836,#181837,#181838,#181839,#181840,
#181841,#181842,#181843,#181844,#181845,#181846,#181847,#181848,#181849,
#181850,#181851,#181852,#181853,#181854,#181855,#181856,#181857,#181858,
#181859,#181860,#181861,#181862,#181863),.UNSPECIFIED.,.F.,.F.,(4,2,2,2,
2,2,2,2,2,2,2,2,2,2,2,2,2,2,2,2,2,2,2,2,2,2,2,2,2,2,2,2,2,2,2,2,2,2,2,2,
2,2,2,2,2,2,2,2,2,2,2,2,2,2,2,2,2,2,2,2,2,2,2,2,2,2,2,2,2,2,2,2,2,2,2,2,
2,2,2,2,2,2,2,2,2,2,2,2,2,4),(-8.95293752943051,-8.94466494354158,-8.92662197800537,
-8.85140677799895,-8.76782829419565,-8.74060822603189,-8.71888012097177,
-8.69221316947022,-8.59829581946537,-8.55954665453933,-8.53363450953526,
-8.52007436829822,-8.50598418094776,-8.47666325842438,-8.40693709867059,
-8.34573803375985,-8.3202210493761,-8.29842109397278,-8.27022466722885,
-8.17852621903307,-8.11350566802394,-8.09609202761019,-8.08443504838779,
-8.06978400359294,-8.03557577626809,-7.9677493481306,-7.90077116864638,
-7.87446608172774,-7.85272892927623,-7.82508518180479,-7.74631650503349,
-7.67782123813631,-7.66117979312411,-7.64854509816135,-7.63268837932748,
-7.54589169709742,-7.49549495842685,-7.46452090650524,-7.44250916966715,
-7.41810679218684,-7.3705817815995,-7.28285829705504,-7.24327831287026,
-7.22841471876788,-7.21678624917497,-7.19969685725232,-7.11505580885114,
-7.06299158652229,-7.02447733489016,-7.00136172911433,-6.97871046342424,
-6.94294481590786,-6.85516535904935,-6.82460801210217,-6.80233839225203,
-6.78933775608357,-6.77428575018232,-6.74244047489071,-6.65967307752173,
-6.62598048187553,-6.59718374005725,-6.57538301579716,-6.54989939096632,
-6.4985783186988,-6.41697460141405,-6.37854004035094,-6.36379609332515,
-6.35215234412663,-6.33488366309922,-6.24073183913631,-6.17215875911867,
-6.14575354115085,-6.12401954842903,-6.09649473247129,-6.014824666104,-5.96989123714106,
-5.949468300581,-5.93259009325537,-5.91997627037338,-5.90435207184409,-5.81614839584029,
-5.76634897365184,-5.73548326381252,-5.71348384115434,-5.68903794321173,
-5.64117931219174,-5.5538610027468,-5.52634787091137,-5.50572248954911,
-5.49514095832648),.UNSPECIFIED.);
#30279=B_SPLINE_CURVE_WITH_KNOTS('',3,(#181864,#181865,#181866,#181867,
#181868,#181869,#181870,#181871,#181872,#181873,#181874,#181875,#181876,
#181877,#181878,#181879,#181880,#181881,#181882,#181883,#181884,#181885,
#181886,#181887,#181888,#181889,#181890,#181891,#181892,#181893,#181894,
#181895,#181896,#181897,#181898,#181899,#181900,#181901,#181902,#181903,
#181904,#181905,#181906,#181907,#181908,#181909,#181910,#181911,#181912,
#181913,#181914,#181915,#181916,#181917,#181918,#181919,#181920,#181921,
#181922,#181923,#181924,#181925,#181926,#181927,#181928,#181929,#181930,
#181931,#181932,#181933,#181934,#181935,#181936,#181937,#181938,#181939,
#181940,#181941,#181942,#181943,#181944,#181945,#181946,#181947,#181948,
#181949,#181950,#181951,#181952,#181953,#181954,#181955,#181956,#181957,
#181958,#181959,#181960,#181961,#181962,#181963,#181964,#181965,#181966,
#181967,#181968,#181969,#181970,#181971,#181972,#181973,#181974,#181975,
#181976,#181977,#181978,#181979,#181980,#181981,#181982,#181983,#181984,
#181985,#181986,#181987,#181988,#181989,#181990,#181991,#181992,#181993,
#181994,#181995,#181996,#181997,#181998,#181999,#182000,#182001,#182002,
#182003,#182004,#182005,#182006,#182007,#182008,#182009,#182010,#182011,
#182012,#182013,#182014,#182015,#182016,#182017,#182018,#182019,#182020,
#182021,#182022,#182023,#182024,#182025,#182026,#182027,#182028,#182029,
#182030,#182031,#182032,#182033,#182034,#182035,#182036,#182037,#182038,
#182039,#182040,#182041),.UNSPECIFIED.,.F.,.F.,(4,2,2,2,2,2,2,2,2,2,2,2,
2,2,2,2,2,2,2,2,2,2,2,2,2,2,2,2,2,2,2,2,2,2,2,2,2,2,2,2,2,2,2,2,2,2,2,2,
2,2,2,2,2,2,2,2,2,2,2,2,2,2,2,2,2,2,2,2,2,2,2,2,2,2,2,2,2,2,2,2,2,2,2,2,
2,2,2,2,4),(-6.16419090700929,-6.15731653447364,-6.14056411527924,-6.05198636916046,
-6.00171152973909,-5.96400099653716,-5.94100788492888,-5.91825471481642,
-5.88177258492111,-5.79423701631445,-5.76426476526426,-5.74227876310545,
-5.729318475769,-5.71416447629465,-5.68167403647096,-5.59960405095324,-5.57696442385519,
-5.5432407280318,-5.52087753886471,-5.49733579815858,-5.45596877366023,
-5.39706516156768,-5.32593660424819,-5.30797910093004,-5.29626443354325,
-5.28193019596578,-5.24705607251649,-5.18119784704434,-5.11376429792051,
-5.08688666352897,-5.06516213418457,-5.03816192426049,-4.96406673182427,
-4.8911901173433,-4.87533543247579,-4.86270167510026,-4.84606012737471,
-4.78147443569736,-4.6983674121006,-4.6708938077729,-4.64916272843381,-4.62271754523909,
-4.55344583906296,-4.46054973531814,-4.44307173244349,-4.43140896996955,
-4.41679899584926,-4.37957931765812,-4.30383060078425,-4.24703356049772,
-4.22094740206581,-4.1994093214977,-4.17162085822899,-4.10513259025917,
-4.02543486564442,-4.00867574916312,-3.99607562882306,-3.97758032318802,
-3.92190701584802,-3.83312939794508,-3.80596068411184,-3.78423510539483,
-3.75751770667088,-3.6826934328211,-3.59484351663941,-3.57798109323278,
-3.56637050500942,-3.55134849971937,-3.51015111117681,-3.41254225725811,
-3.37251827322652,-3.34917679648139,-3.32669312229479,-3.29209838160418,
-3.24721117712543,-3.1596699041009,-3.14330180894059,-3.13063545158538,
-3.11115330335491,-3.08608005778132,-3.01605958134592,-2.96332610827766,
-2.93796238003775,-2.91614401066078,-2.88720122760286,-2.81504547153266,
-2.73079590200839,-2.71376506241483,-2.70657200810638),.UNSPECIFIED.);
#30280=B_SPLINE_CURVE_WITH_KNOTS('',3,(#182046,#182047,#182048,#182049,
#182050,#182051,#182052,#182053,#182054,#182055,#182056,#182057,#182058,
#182059,#182060,#182061,#182062,#182063),.UNSPECIFIED.,.F.,.F.,(4,2,2,2,
2,2,2,2,4),(3.80158966705551,3.91441070971229,4.3189896343053,4.69887283496923,
5.04702075342428,5.38197377559302,5.74008106147176,5.97805601036782,6.26584118659148),
 .UNSPECIFIED.);
#30281=B_SPLINE_CURVE_WITH_KNOTS('',3,(#182070,#182071,#182072,#182073,
#182074,#182075,#182076,#182077,#182078,#182079,#182080,#182081,#182082,
#182083,#182084,#182085,#182086,#182087,#182088,#182089,#182090,#182091,
#182092,#182093,#182094,#182095,#182096,#182097,#182098,#182099,#182100,
#182101,#182102,#182103,#182104,#182105,#182106,#182107,#182108,#182109,
#182110,#182111,#182112,#182113,#182114,#182115,#182116,#182117,#182118,
#182119,#182120,#182121,#182122,#182123,#182124,#182125,#182126,#182127,
#182128,#182129,#182130,#182131,#182132,#182133,#182134,#182135,#182136,
#182137,#182138,#182139,#182140,#182141,#182142,#182143,#182144,#182145,
#182146,#182147),.UNSPECIFIED.,.F.,.F.,(4,2,2,2,2,2,2,2,2,2,2,2,2,2,2,2,
2,2,2,2,2,2,2,2,2,2,2,2,2,2,2,2,2,2,2,2,2,2,4),(6.88948415565909,6.89141801458342,
6.90474021311763,6.93177588713481,6.97221514823743,7.08776936697473,7.11769020949234,
7.13962540316573,7.16415849604642,7.21203763277651,7.29039380168267,7.33921802785112,
7.35560423878488,7.36816059809641,7.3862691115726,7.45046823029671,7.54624104871021,
7.57432106142301,7.59611687794412,7.62140064381964,7.67372768818048,7.76255670421757,
7.81014142349575,7.82459371238885,7.83623675695614,7.85051909614518,7.88377441630314,
7.94084361064966,8.02992242379317,8.06017844583965,8.08215257062765,8.10653377932961,
8.15328396329187,8.22131431393986,8.27667423996549,8.29572185013062,8.30814872058125,
8.32014034829938,8.34523528310529),.UNSPECIFIED.);
#30282=B_SPLINE_CURVE_WITH_KNOTS('',3,(#182150,#182151,#182152,#182153,
#182154,#182155,#182156,#182157,#182158,#182159,#182160,#182161,#182162,
#182163,#182164,#182165,#182166,#182167,#182168,#182169,#182170,#182171,
#182172,#182173,#182174,#182175,#182176,#182177,#182178,#182179,#182180,
#182181,#182182,#182183,#182184,#182185,#182186,#182187,#182188,#182189,
#182190,#182191,#182192,#182193,#182194,#182195,#182196,#182197,#182198,
#182199,#182200,#182201,#182202,#182203,#182204,#182205),.UNSPECIFIED.,
 .F.,.F.,(4,2,2,2,2,2,2,2,2,2,2,2,2,2,2,2,2,2,2,2,2,2,2,2,2,2,2,4),(1.00000001712619E-6,
0.0947119972862606,0.109535172509233,0.122857363566205,0.134658169476671,
0.153906771232427,0.234207439936081,0.296649708059561,0.340368572332069,
0.364427318761554,0.386499398388915,0.412681983689554,0.517013231527544,
0.57373595734596,0.590623080685259,0.603169022656912,0.621031899335483,
0.711114334859672,0.785685359291965,0.812534065126885,0.834250299145937,
0.86086282768967,0.920548379689519,0.926540857549104,1.0078403703309,1.04760215944455,
1.0626981323893,1.06776182258593),.UNSPECIFIED.);
#30283=B_SPLINE_CURVE_WITH_KNOTS('',3,(#182210,#182211,#182212,#182213,
#182214,#182215,#182216,#182217,#182218,#182219,#182220,#182221,#182222,
#182223,#182224,#182225,#182226,#182227,#182228,#182229,#182230,#182231,
#182232,#182233,#182234,#182235,#182236,#182237,#182238,#182239,#182240,
#182241,#182242,#182243,#182244,#182245,#182246,#182247,#182248,#182249,
#182250,#182251,#182252,#182253,#182254,#182255,#182256,#182257,#182258,
#182259,#182260,#182261,#182262,#182263,#182264,#182265,#182266,#182267,
#182268,#182269,#182270,#182271,#182272,#182273,#182274,#182275,#182276,
#182277,#182278,#182279,#182280,#182281,#182282,#182283,#182284,#182285,
#182286,#182287,#182288,#182289,#182290,#182291,#182292,#182293,#182294,
#182295,#182296,#182297,#182298,#182299,#182300,#182301,#182302,#182303,
#182304,#182305,#182306,#182307,#182308,#182309,#182310,#182311,#182312,
#182313,#182314,#182315,#182316,#182317,#182318,#182319,#182320,#182321,
#182322,#182323,#182324,#182325,#182326,#182327,#182328,#182329,#182330,
#182331,#182332,#182333,#182334,#182335,#182336,#182337,#182338,#182339,
#182340,#182341,#182342,#182343,#182344,#182345,#182346,#182347,#182348,
#182349,#182350,#182351,#182352,#182353,#182354,#182355,#182356,#182357,
#182358,#182359,#182360,#182361,#182362,#182363,#182364,#182365,#182366,
#182367,#182368,#182369,#182370,#182371,#182372,#182373,#182374,#182375,
#182376,#182377,#182378,#182379,#182380,#182381,#182382,#182383,#182384,
#182385,#182386,#182387,#182388,#182389,#182390,#182391,#182392,#182393,
#182394,#182395,#182396,#182397,#182398,#182399),.UNSPECIFIED.,.F.,.F.,
(4,2,2,2,2,2,2,2,2,2,2,2,2,2,2,2,2,2,2,2,2,2,2,2,2,2,2,2,2,2,2,2,2,2,2,
2,2,2,2,2,2,2,2,2,2,2,2,2,2,2,2,2,2,2,2,2,2,2,2,2,2,2,2,2,2,2,2,2,2,2,2,
2,2,2,2,2,2,2,2,2,2,2,2,2,2,2,2,2,2,2,2,2,2,2,4),(3.11744395882936,3.12694151309502,
3.14579754015536,3.24459640843926,3.30628076311852,3.34053666865373,3.36308156246976,
3.38623505328776,3.42464055749654,3.5202847142483,3.56776294756924,3.58408491513238,
3.59667182302396,3.61220276931054,3.67683258823788,3.74351999935887,3.7877598262854,
3.81179123517777,3.83387831942606,3.86004480977197,3.96913524517012,4.01490588650292,
4.04412676213954,4.05780824464263,4.06947278689076,4.08782109592327,4.17268601614708,
4.25777089488721,4.28810886071105,4.31009463674667,4.33444400400631,4.38094817055307,
4.45459771554067,4.50649591984476,4.52470157414305,4.5372638493657,4.55387211568767,
4.60544171108894,4.72285039684045,4.74921521875177,4.76876842552846,4.79477459882673,
4.85313308550783,4.97268136874961,4.9928818035547,5.00377846445466,5.01636385097906,
5.03928727157169,5.07083044565121,5.13298455450813,5.20705851567379,5.23460909473655,
5.25637191982548,5.2820048772336,5.33933355425583,5.41053597534993,5.4515007565642,
5.46715927407271,5.47976014339252,5.49596056164844,5.54191540591792,5.64133736785147,
5.67866939863431,5.70165617682956,5.72433342209488,5.75942599766235,5.80332579814885,
5.87225678500807,5.92345674406103,5.93979175548642,5.95135294957844,5.96627996610724,
6.00455883449701,6.07943996231504,6.15042525690114,6.17811953207395,6.19986266661448,
6.22573949973217,6.28563697419499,6.35590403733274,6.39677568424294,6.41294399314959,
6.42551768899698,6.44392129981866,6.46673152154306,6.52040099614958,6.60158366471143,
6.62777382705719,6.64984804132894,6.67390457814773,6.71760477527127,6.77999880564105,
6.86036549578554,6.87961643495318,6.88948415565909),.UNSPECIFIED.);
#30284=B_SPLINE_CURVE_WITH_KNOTS('',3,(#182400,#182401,#182402,#182403,
#182404,#182405,#182406,#182407,#182408,#182409,#182410,#182411,#182412,
#182413,#182414,#182415,#182416,#182417,#182418,#182419,#182420,#182421,
#182422,#182423,#182424,#182425,#182426,#182427,#182428,#182429,#182430,
#182431,#182432,#182433,#182434,#182435,#182436,#182437,#182438,#182439,
#182440,#182441,#182442,#182443,#182444,#182445,#182446,#182447,#182448,
#182449,#182450,#182451,#182452,#182453,#182454,#182455,#182456,#182457,
#182458,#182459,#182460,#182461,#182462,#182463,#182464,#182465,#182466,
#182467,#182468,#182469,#182470,#182471,#182472,#182473,#182474,#182475,
#182476,#182477,#182478,#182479,#182480,#182481,#182482,#182483,#182484,
#182485,#182486,#182487,#182488,#182489,#182490,#182491,#182492,#182493,
#182494,#182495,#182496,#182497,#182498,#182499,#182500,#182501,#182502,
#182503,#182504,#182505,#182506,#182507,#182508,#182509,#182510,#182511,
#182512,#182513,#182514,#182515,#182516,#182517,#182518,#182519,#182520,
#182521,#182522,#182523,#182524,#182525,#182526,#182527,#182528,#182529,
#182530,#182531,#182532,#182533,#182534,#182535,#182536,#182537,#182538,
#182539,#182540,#182541,#182542,#182543,#182544,#182545,#182546,#182547,
#182548,#182549,#182550,#182551,#182552,#182553,#182554,#182555,#182556,
#182557,#182558,#182559,#182560,#182561,#182562,#182563,#182564,#182565,
#182566,#182567,#182568,#182569,#182570,#182571,#182572,#182573,#182574,
#182575,#182576,#182577,#182578,#182579,#182580,#182581,#182582,#182583,
#182584,#182585,#182586,#182587),.UNSPECIFIED.,.F.,.F.,(4,2,2,2,2,2,2,2,
2,2,2,2,2,2,2,2,2,2,2,2,2,2,2,2,2,2,2,2,2,2,2,2,2,2,2,2,2,2,2,2,2,2,2,2,
2,2,2,2,2,2,2,2,2,2,2,2,2,2,2,2,2,2,2,2,2,2,2,2,2,2,2,2,2,2,2,2,2,2,2,2,
2,2,2,2,2,2,2,2,2,2,2,2,2,4),(1.06776182258593,1.07424788354723,1.09037184154246,
1.13945079036451,1.2270035492851,1.27899909195985,1.30424012793862,1.32604164394563,
1.3541890587477,1.44889705400479,1.51321247283617,1.53167700348148,1.54425451446089,
1.56037901360682,1.60109455708781,1.67451960508606,1.73219945160084,1.75786609105852,
1.77962428141715,1.80712543760684,1.88626840594513,1.95481635508634,1.99147171609752,
2.00620231139152,2.01778094040984,2.03437793173402,2.08423345261758,2.17045781598089,
2.22209877833376,2.24729351920513,2.26910145791718,2.29732302490004,2.39064538694898,
2.45651016745175,2.47480704713921,2.48737389968575,2.50361875572393,2.54471688484202,
2.61843298859145,2.67537943962706,2.70097303378857,2.72273790630625,2.75033781881128,
2.8680181519061,2.91025725622607,2.93805260894651,2.95150230303917,2.96324978649333,
2.9821578899495,3.08066359977336,3.14194758412427,3.17649896256903,3.19909030348181,
3.22218229194078,3.26019178363487,3.36213004842725,3.40501331314863,3.42094058353768,
3.43357995091236,3.45277606974348,3.51769337946013,3.58144858110792,3.60200392198475,
3.63399817820798,3.65618344693286,3.67996223747849,3.72188229728814,3.83069624635579,
3.87536641780213,3.8909616664111,3.90249964789073,3.9178018861172,3.95775315380778,
4.02782764509861,4.07794464122129,4.11619913461445,4.13938862233777,4.16164538356313,
4.1956754392536,4.23845769308302,4.34315482837855,4.36118053643026,4.37373407659236,
4.39048715927313,4.44452015701052,4.5586118465161,4.58514890648456,4.60686784061629,
4.63379679261957,4.70191902674089,4.771251252303,4.81766625531918,4.83203831894305,
4.83979364673243),.UNSPECIFIED.);
#30285=B_SPLINE_CURVE_WITH_KNOTS('',3,(#182614,#182615,#182616,#182617,
#182618,#182619,#182620,#182621,#182622,#182623),.UNSPECIFIED.,.F.,.F.,
(4,3,3,4),(0.,0.466042421267126,0.940249856436761,1.),.UNSPECIFIED.);
#30286=B_SPLINE_CURVE_WITH_KNOTS('',3,(#182635,#182636,#182637,#182638,
#182639,#182640,#182641,#182642,#182643,#182644,#182645,#182646,#182647,
#182648,#182649,#182650,#182651,#182652,#182653,#182654,#182655,#182656,
#182657,#182658,#182659,#182660,#182661,#182662,#182663,#182664,#182665,
#182666,#182667,#182668,#182669,#182670,#182671,#182672,#182673,#182674,
#182675,#182676,#182677,#182678,#182679,#182680,#182681,#182682,#182683,
#182684,#182685,#182686,#182687,#182688,#182689,#182690,#182691,#182692,
#182693,#182694,#182695,#182696,#182697,#182698,#182699,#182700,#182701,
#182702,#182703,#182704,#182705,#182706,#182707,#182708,#182709,#182710,
#182711,#182712,#182713,#182714,#182715,#182716,#182717,#182718,#182719,
#182720,#182721,#182722,#182723,#182724,#182725,#182726,#182727,#182728,
#182729,#182730,#182731,#182732,#182733,#182734,#182735,#182736,#182737,
#182738,#182739,#182740,#182741,#182742,#182743,#182744,#182745,#182746,
#182747,#182748,#182749,#182750,#182751,#182752,#182753,#182754,#182755,
#182756,#182757,#182758,#182759,#182760,#182761,#182762,#182763,#182764,
#182765,#182766,#182767,#182768,#182769,#182770,#182771,#182772,#182773,
#182774,#182775,#182776,#182777,#182778,#182779,#182780,#182781,#182782,
#182783,#182784,#182785,#182786,#182787,#182788,#182789,#182790,#182791,
#182792,#182793,#182794,#182795,#182796,#182797,#182798,#182799,#182800,
#182801,#182802,#182803,#182804,#182805,#182806,#182807,#182808,#182809,
#182810),.UNSPECIFIED.,.F.,.F.,(4,2,2,2,2,2,2,2,2,2,2,2,2,2,2,2,2,2,2,2,
2,2,2,2,2,2,2,2,2,2,2,2,2,2,2,2,2,2,2,2,2,2,2,2,2,2,2,2,2,2,2,2,2,2,2,2,
2,2,2,2,2,2,2,2,2,2,2,2,2,2,2,2,2,2,2,2,2,2,2,2,2,2,2,2,2,2,2,4),(4.83979364673243,
4.84367014322603,4.85802029975688,4.89176076265798,4.9503386380513,5.03714167429101,
5.06744736122364,5.0894287373729,5.11379099582578,5.16039299666449,5.23436606903538,
5.28708932448838,5.30469658181848,5.31723609741978,5.33435263414912,5.3971999728895,
5.49763805243059,5.52530333933724,5.54706898097428,5.57263536588406,5.62720509399079,
5.72548818007443,5.76272841944928,5.77763157651974,5.78917837969072,5.80522127391578,
5.85530303480364,5.95717195261677,5.99938153238094,6.02320564045918,6.04537037249978,
6.07721790956922,6.09763102156905,6.16061416364242,6.22686448743711,6.24599901729141,
6.25863210695444,6.274596068554,6.31787131798,6.42250893271361,6.45878788619945,
6.48161023218432,6.50443757194009,6.54046997542785,6.58616209400338,6.65534263176113,
6.70335009057412,6.71783260264344,6.72948023359561,6.74373813814339,6.77681903931524,
6.83335381360029,6.9232754924118,6.95350270842544,6.97547332750822,6.99986701859546,
7.04670943674406,7.12148632426097,7.17495111535607,7.19154073776591,7.20408600217487,
7.22193927577781,7.2437988308098,7.29316361060375,7.38155535794701,7.40997901253632,
7.43180435601276,7.45687485781199,7.5075866571292,7.59047867266803,7.64469907080788,
7.66142826971883,7.67301707905495,7.68765387073351,7.72356600357138,7.78941553209505,
7.86553410640628,7.89603339619037,7.91803699914874,7.94231427265443,7.98830867777345,
8.06032117887829,8.11302803706241,8.13198929278981,8.14460558454549,8.16067628809637,
8.2051332456036,8.32330225647707),.UNSPECIFIED.);
#30287=B_SPLINE_CURVE_WITH_KNOTS('',3,(#182813,#182814,#182815,#182816,
#182817,#182818,#182819,#182820,#182821,#182822,#182823,#182824,#182825,
#182826,#182827,#182828,#182829,#182830,#182831,#182832,#182833,#182834,
#182835,#182836,#182837,#182838,#182839,#182840,#182841,#182842,#182843,
#182844,#182845,#182846,#182847,#182848,#182849,#182850,#182851,#182852,
#182853,#182854,#182855,#182856,#182857,#182858,#182859,#182860,#182861,
#182862,#182863,#182864,#182865,#182866,#182867,#182868,#182869,#182870,
#182871,#182872,#182873,#182874,#182875,#182876,#182877,#182878,#182879,
#182880,#182881,#182882,#182883,#182884,#182885,#182886,#182887,#182888,
#182889,#182890,#182891,#182892,#182893,#182894,#182895,#182896,#182897,
#182898,#182899,#182900,#182901,#182902,#182903,#182904,#182905,#182906,
#182907,#182908,#182909,#182910,#182911,#182912,#182913,#182914,#182915,
#182916,#182917,#182918,#182919,#182920,#182921,#182922,#182923,#182924,
#182925,#182926,#182927,#182928,#182929,#182930,#182931,#182932,#182933,
#182934,#182935,#182936,#182937,#182938,#182939,#182940,#182941,#182942,
#182943,#182944,#182945,#182946,#182947,#182948,#182949,#182950,#182951,
#182952,#182953,#182954,#182955,#182956,#182957,#182958,#182959,#182960,
#182961,#182962,#182963,#182964,#182965,#182966,#182967,#182968,#182969,
#182970,#182971,#182972),.UNSPECIFIED.,.F.,.F.,(4,2,2,2,2,2,2,2,2,2,2,2,
2,2,2,2,2,2,2,2,2,2,2,2,2,2,2,2,2,2,2,2,2,2,2,2,2,2,2,2,2,2,2,2,2,2,2,2,
2,2,2,2,2,2,2,2,2,2,2,2,2,2,2,2,2,2,2,2,2,2,2,2,2,2,2,2,2,2,2,4),(0.000225337909139367,
0.0292717095416562,0.0505239070880682,0.0751504710126493,0.119984405057097,
0.222628091878377,0.267192334550033,0.282776676146931,0.294313533193336,
0.309623314590521,0.349645533055194,0.419702387883073,0.476031974073537,
0.510940415084872,0.533587424214121,0.556607355965541,0.594159068655156,
0.690053826025381,0.738607405494358,0.755009621309299,0.767587828478025,
0.78303625440397,0.832973737062743,0.909671379078525,0.957079771885631,
0.981550402261636,1.00350136931844,1.03355831363916,1.14829431806412,1.1890215181048,
1.21618042059942,1.22952351576019,1.24131581869561,1.26050889790246,1.34195804753588,
1.43121477359485,1.46053881398604,1.4824100984169,1.50724122817928,1.55743393075515,
1.5783724429731,1.64795120208137,1.67372298916354,1.6937833995583,1.70651884828274,
1.72197251917669,1.75543462582521,1.82719833229392,1.89367459809474,1.92007460444182,
1.94179461045165,1.96886675656026,2.03221009135532,2.11430237212839,2.15423737604396,
2.16935263342085,2.18090146087354,2.19700260542734,2.24578624585707,2.33359222314304,
2.38565465677845,2.41090453658282,2.43270506830581,2.46083903427388,2.55577376470094,
2.61990655913048,2.63836773569775,2.65094509986822,2.66707215988022,2.71091140333411,
2.78317198810242,2.83937087960711,2.86488791011897,2.88666018259058,2.91436577524644,
3.03128114050773,3.07381474163023,3.10173217448532,3.11520207107795,3.11744395882936),
 .UNSPECIFIED.);
#30288=B_SPLINE_CURVE_WITH_KNOTS('',3,(#182976,#182977,#182978,#182979,
#182980,#182981),.UNSPECIFIED.,.F.,.F.,(4,2,4),(1.45420179664634,1.60034795961777,
1.7792155245964),.UNSPECIFIED.);
#30289=B_SPLINE_CURVE_WITH_KNOTS('',3,(#182985,#182986,#182987,#182988,
#182989,#182990,#182991,#182992,#182993,#182994,#182995,#182996,#182997,
#182998,#182999,#183000,#183001,#183002,#183003,#183004,#183005,#183006,
#183007,#183008,#183009,#183010),.UNSPECIFIED.,.F.,.F.,(4,2,2,2,2,2,2,2,
2,2,2,2,4),(1.00000001384073E-6,0.147496320872454,0.27627744997771,0.416495853131057,
0.550555574701638,0.664844786569313,0.796386308624163,0.911514817984701,
1.04112230610171,1.1590206206347,1.29683959014132,1.43253712595453,1.45420179664634),
 .UNSPECIFIED.);
#30290=B_SPLINE_CURVE_WITH_KNOTS('',3,(#183034,#183035,#183036,#183037,
#183038,#183039,#183040,#183041),.UNSPECIFIED.,.F.,.F.,(4,2,2,4),(-0.422074901515015,
-0.379068128351578,-0.282387357989601,-0.250738867764476),.UNSPECIFIED.);
#30291=B_SPLINE_CURVE_WITH_KNOTS('',3,(#183046,#183047,#183048,#183049,
#183050,#183051,#183052),.UNSPECIFIED.,.F.,.F.,(4,3,4),(-0.0851792640752978,
0.,0.0851792640752318),.UNSPECIFIED.);
#30292=B_SPLINE_CURVE_WITH_KNOTS('',3,(#183059,#183060,#183061,#183062,
#183063,#183064,#183065,#183066,#183067,#183068,#183069,#183070,#183071,
#183072,#183073,#183074,#183075),.UNSPECIFIED.,.F.,.F.,(4,2,2,2,1,2,2,2,
4),(0.691841692846147,0.730361481240391,0.749621375437511,0.754436348986791,
0.759251322536071,0.768881269634628,0.845920846423085,0.922960423211543,
1.),.UNSPECIFIED.);
#30293=B_SPLINE_CURVE_WITH_KNOTS('',3,(#183076,#183077,#183078,#183079,
#183080,#183081,#183082,#183083,#183084,#183085,#183086,#183087,#183088,
#183089,#183090,#183091,#183092,#183093,#183094,#183095,#183096,#183097,
#183098,#183099,#183100,#183101,#183102,#183103,#183104,#183105,#183106,
#183107,#183108,#183109,#183110,#183111,#183112,#183113,#183114,#183115,
#183116,#183117,#183118,#183119,#183120,#183121,#183122,#183123,#183124,
#183125,#183126,#183127,#183128,#183129,#183130,#183131,#183132,#183133,
#183134,#183135,#183136,#183137,#183138,#183139,#183140,#183141,#183142,
#183143,#183144,#183145,#183146,#183147,#183148,#183149,#183150,#183151,
#183152,#183153,#183154,#183155,#183156,#183157,#183158,#183159,#183160),
 .UNSPECIFIED.,.F.,.F.,(4,3,3,3,3,3,3,3,3,3,3,3,3,3,3,3,3,3,3,3,3,3,3,3,
3,3,3,3,4),(0.,0.0480329457521728,0.0955923583820344,0.142452410367028,
0.172960423211526,0.227007917172798,0.280795071156351,0.334180568678605,
0.345920846423051,0.391773667569033,0.432401058028814,0.475641163831695,
0.497261216733136,0.502746609445371,0.508071243183858,0.51888126963458,
0.542844921349788,0.567150056988716,0.591940455940715,0.605361481240375,
0.616171507691099,0.621576520916459,0.624279027529142,0.626981534141824,
0.642242401576597,0.648601587043266,0.663892977132314,0.679172488710331,
0.691841689138341),.UNSPECIFIED.);
#30294=B_SPLINE_CURVE_WITH_KNOTS('',3,(#183161,#183162,#183163,#183164,
#183165,#183166,#183167,#183168,#183169,#183170,#183171,#183172,#183173,
#183174,#183175,#183176,#183177,#183178,#183179,#183180,#183181,#183182,
#183183,#183184),.UNSPECIFIED.,.F.,.F.,(4,2,2,2,2,2,2,2,2,2,2,4),(1.00000001309674E-6,
0.129224229604342,0.241263601967655,0.496076308060944,0.797054408048329,
1.12551872852194,1.51457617341985,1.9211054184316,2.48023648950879,2.94600632909222,
3.4283141418049,3.80158966705551),.UNSPECIFIED.);
#30295=B_SPLINE_CURVE_WITH_KNOTS('',3,(#183190,#183191,#183192,#183193,
#183194,#183195,#183196,#183197,#183198,#183199,#183200,#183201,#183202,
#183203,#183204,#183205,#183206,#183207,#183208,#183209,#183210,#183211,
#183212,#183213,#183214,#183215,#183216,#183217,#183218,#183219,#183220,
#183221,#183222,#183223,#183224,#183225,#183226,#183227,#183228,#183229,
#183230,#183231,#183232,#183233,#183234,#183235,#183236,#183237,#183238,
#183239,#183240,#183241,#183242,#183243,#183244,#183245,#183246,#183247,
#183248,#183249,#183250,#183251,#183252,#183253,#183254,#183255,#183256,
#183257,#183258,#183259,#183260,#183261,#183262,#183263,#183264,#183265,
#183266,#183267,#183268,#183269,#183270,#183271,#183272,#183273,#183274,
#183275,#183276,#183277,#183278,#183279,#183280,#183281,#183282,#183283,
#183284,#183285,#183286,#183287,#183288,#183289,#183290,#183291,#183292,
#183293,#183294,#183295,#183296,#183297,#183298,#183299,#183300,#183301,
#183302,#183303,#183304,#183305,#183306,#183307,#183308,#183309,#183310,
#183311,#183312,#183313,#183314,#183315,#183316,#183317,#183318,#183319,
#183320,#183321,#183322,#183323,#183324,#183325,#183326,#183327,#183328,
#183329,#183330,#183331,#183332,#183333),.UNSPECIFIED.,.F.,.F.,(4,2,2,2,
2,2,2,2,2,2,2,2,2,2,2,2,2,2,2,2,2,2,2,2,2,2,2,2,2,2,2,2,2,2,2,2,2,2,2,2,
2,2,2,2,2,2,2,2,2,2,2,2,2,2,2,2,2,2,2,2,2,2,2,2,2,2,2,2,2,2,2,4),(-2.70657200810638,
-2.70214184710763,-2.68723936465603,-2.64726736463653,-2.55727944885561,
-2.51159438667173,-2.48743895240915,-2.46534998566859,-2.43371879553524,
-2.41324657383308,-2.34693664433086,-2.29546775853098,-2.27919589566977,
-2.26667452046651,-2.24761514929512,-2.22332511326117,-2.15842203129561,
-2.100283970418,-2.07450170525313,-2.05272929755366,-2.02442294882669,-1.95492881376122,
-1.86554060462523,-1.84891352543864,-1.83731748462922,-1.82211690291699,
-1.77896342050705,-1.66685971268145,-1.63563287714678,-1.6135740399562,
-1.58931660936387,-1.541621602447,-1.45740584130219,-1.42569639648637,-1.41126743469913,
-1.39795078874467,-1.37357931312205,-1.30288363529104,-1.23665700931164,
-1.2106035121226,-1.1888514958355,-1.16091132341498,-1.12915158688185,-1.06214283552152,
-1.00473805161412,-0.98636319840359,-0.974597196061126,-0.960477052669798,
-0.927287673755786,-0.867607488061156,-0.797545140108554,-0.768454686778253,
-0.746624285458318,-0.721349851053767,-0.663411959843093,-0.568693706683454,
-0.553023634158854,-0.54040672331115,-0.523578440895917,-0.503240896751126,
-0.45867043084094,-0.376406353474949,-0.348904053221221,-0.327171805956353,
-0.300750127078341,-0.231888909936616,-0.138442844373473,-0.120995821362398,
-0.109335903594524,-0.0947063495243196,-0.0748468037826614,-1.00000001657108E-6),
 .UNSPECIFIED.);
#30296=B_SPLINE_CURVE_WITH_KNOTS('',3,(#183334,#183335,#183336,#183337,
#183338,#183339,#183340,#183341,#183342,#183343,#183344,#183345,#183346,
#183347,#183348,#183349,#183350,#183351,#183352,#183353,#183354,#183355,
#183356,#183357,#183358,#183359,#183360,#183361,#183362,#183363,#183364,
#183365,#183366,#183367,#183368,#183369,#183370,#183371,#183372,#183373,
#183374,#183375,#183376,#183377,#183378,#183379,#183380,#183381,#183382,
#183383,#183384,#183385,#183386,#183387,#183388,#183389,#183390,#183391,
#183392,#183393,#183394,#183395,#183396,#183397,#183398,#183399,#183400,
#183401,#183402,#183403,#183404,#183405,#183406,#183407,#183408,#183409,
#183410,#183411,#183412,#183413,#183414,#183415,#183416,#183417,#183418,
#183419,#183420,#183421,#183422,#183423,#183424,#183425,#183426,#183427,
#183428,#183429,#183430,#183431,#183432,#183433,#183434,#183435,#183436,
#183437,#183438,#183439,#183440,#183441,#183442,#183443),.UNSPECIFIED.,
 .F.,.F.,(4,2,2,2,2,2,2,2,2,2,2,2,2,2,2,2,2,2,2,2,2,2,2,2,2,2,2,2,2,2,2,
2,2,2,2,2,2,2,2,2,2,2,2,2,2,2,2,2,2,2,2,2,2,2,4),(-11.0525898219334,-10.9451955405454,
-10.9175376166771,-10.8958004433713,-10.8695079718537,-10.8058361867022,
-10.7358477644187,-10.6999437907365,-10.6854850563783,-10.6737953686814,
-10.6560609945434,-10.5646795309562,-10.4945715412295,-10.468079086281,
-10.446348643571,-10.4189280801612,-10.33433506663,-10.2718010737687,-10.2548428267076,
-10.2422351870229,-10.2266867142584,-10.144336853529,-10.0977280708593,
-10.0810002635724,-10.0532562691983,-10.0315155882965,-10.0052916010387,
-9.94867170022827,-9.8730873610219,-9.83590140699322,-9.82129460438642,
-9.80963062924863,-9.79214544329891,-9.7116523592644,-9.63517351316824,
-9.60684048441813,-9.58506591829065,-9.55930136163698,-9.5022068778219,
-9.43646311463777,-9.41203817947794,-9.39290563146559,-9.3803783558284,
-9.3641536887642,-9.30976579535966,-9.24532094133244,-9.21469225226209,
-9.18765718227209,-9.16593182042167,-9.13908611089903,-9.06964232827476,
-9.00518783627803,-8.97067935807782,-8.95639002715814,-8.95293752943051),
 .UNSPECIFIED.);
#30297=B_SPLINE_CURVE_WITH_KNOTS('',3,(#183732,#183733,#183734,#183735,
#183736,#183737,#183738,#183739,#183740,#183741),.UNSPECIFIED.,.F.,.F.,
(4,3,3,4),(0.,0.466042421235165,0.94024985640319,1.),.UNSPECIFIED.);
#31337=CIRCLE('',#80850,2.05000000000001);
#31338=CIRCLE('',#80851,2.05);
#31339=CIRCLE('',#80852,2.05);
#31340=CIRCLE('',#80856,5.5);
#31341=CIRCLE('',#80860,5.5);
#31342=CIRCLE('',#80862,6.);
#31343=CIRCLE('',#80865,7.);
#31344=CIRCLE('',#80866,7.);
#31345=CIRCLE('',#80867,7.);
#31346=CIRCLE('',#80868,7.);
#31347=CIRCLE('',#80869,7.);
#31348=CIRCLE('',#80870,7.);
#31349=CIRCLE('',#80872,6.5);
#31350=CIRCLE('',#80874,5.25);
#31351=CIRCLE('',#80875,5.25);
#31352=CIRCLE('',#80877,6.);
#31353=CIRCLE('',#80879,5.5);
#31354=CIRCLE('',#80880,155.44481082364);
#31355=CIRCLE('',#80882,4.4);
#31356=CIRCLE('',#80883,4.4);
#31357=CIRCLE('',#80884,4.4);
#31358=CIRCLE('',#80886,2.55);
#31359=CIRCLE('',#80887,2.55);
#31360=CIRCLE('',#80888,2.55);
#31361=CIRCLE('',#80889,2.55);
#31362=CIRCLE('',#80891,3.05);
#31363=CIRCLE('',#80893,3.05);
#31364=CIRCLE('',#80895,5.5);
#31365=CIRCLE('',#80897,4.9);
#31366=CIRCLE('',#80900,6.47238979616113);
#31367=CIRCLE('',#80901,6.47238979616116);
#31368=CIRCLE('',#80903,0.959420631745662);
#31369=CIRCLE('',#80904,6.47238979616113);
#31370=CIRCLE('',#80906,6.47238979616113);
#31371=CIRCLE('',#80908,9.);
#31372=CIRCLE('',#80909,9.);
#31373=CIRCLE('',#80910,9.);
#31374=CIRCLE('',#80912,9.99999999999999);
#31375=CIRCLE('',#80913,10.);
#31376=CIRCLE('',#80914,10.);
#31377=CIRCLE('',#80916,9.49999999999999);
#31378=CIRCLE('',#80917,0.5);
#31379=CIRCLE('',#80919,9.50000000000001);
#31380=CIRCLE('',#80920,0.5);
#31381=CIRCLE('',#80922,0.5);
#31382=CIRCLE('',#80924,7.99999999999999);
#31383=CIRCLE('',#80925,7.99999999999999);
#31384=CIRCLE('',#80927,0.5);
#31385=CIRCLE('',#80928,7.5);
#31386=CIRCLE('',#80930,4.);
#31387=CIRCLE('',#80931,4.);
#31388=CIRCLE('',#80933,2.30850939467147);
#31389=CIRCLE('',#80934,2.30850939467147);
#31390=CIRCLE('',#80949,6.5);
#34941=VERTEX_POINT('',#181112);
#34942=VERTEX_POINT('',#181114);
#34943=VERTEX_POINT('',#181116);
#34944=VERTEX_POINT('',#181120);
#34945=VERTEX_POINT('',#181124);
#34946=VERTEX_POINT('',#181125);
#34947=VERTEX_POINT('',#181127);
#34948=VERTEX_POINT('',#181238);
#34949=VERTEX_POINT('',#181317);
#34950=VERTEX_POINT('',#181318);
#34951=VERTEX_POINT('',#181681);
#34952=VERTEX_POINT('',#181682);
#34953=VERTEX_POINT('',#182043);
#34954=VERTEX_POINT('',#182044);
#34955=VERTEX_POINT('',#182066);
#34956=VERTEX_POINT('',#182067);
#34957=VERTEX_POINT('',#182069);
#34958=VERTEX_POINT('',#182148);
#34959=VERTEX_POINT('',#182207);
#34960=VERTEX_POINT('',#182208);
#34961=VERTEX_POINT('',#182589);
#34962=VERTEX_POINT('',#182591);
#34963=VERTEX_POINT('',#182593);
#34964=VERTEX_POINT('',#182595);
#34965=VERTEX_POINT('',#182597);
#34966=VERTEX_POINT('',#182599);
#34967=VERTEX_POINT('',#182601);
#34968=VERTEX_POINT('',#182603);
#34969=VERTEX_POINT('',#182605);
#34970=VERTEX_POINT('',#182607);
#34971=VERTEX_POINT('',#182611);
#34972=VERTEX_POINT('',#182612);
#34973=VERTEX_POINT('',#182628);
#34974=VERTEX_POINT('',#182630);
#34975=VERTEX_POINT('',#182634);
#34976=VERTEX_POINT('',#182811);
#34977=VERTEX_POINT('',#182974);
#34978=VERTEX_POINT('',#182975);
#34979=VERTEX_POINT('',#182982);
#34980=VERTEX_POINT('',#183013);
#34981=VERTEX_POINT('',#183014);
#34982=VERTEX_POINT('',#183016);
#34983=VERTEX_POINT('',#183021);
#34984=VERTEX_POINT('',#183022);
#34985=VERTEX_POINT('',#183024);
#34986=VERTEX_POINT('',#183026);
#34987=VERTEX_POINT('',#183028);
#34988=VERTEX_POINT('',#183030);
#34989=VERTEX_POINT('',#183042);
#34990=VERTEX_POINT('',#183053);
#34991=VERTEX_POINT('',#183058);
#34992=VERTEX_POINT('',#183186);
#34993=VERTEX_POINT('',#183445);
#34994=VERTEX_POINT('',#183447);
#34995=VERTEX_POINT('',#183451);
#34996=VERTEX_POINT('',#183455);
#34997=VERTEX_POINT('',#183459);
#34998=VERTEX_POINT('',#183460);
#34999=VERTEX_POINT('',#183462);
#35000=VERTEX_POINT('',#183467);
#35001=VERTEX_POINT('',#183469);
#35002=VERTEX_POINT('',#183471);
#35003=VERTEX_POINT('',#183475);
#35004=VERTEX_POINT('',#183479);
#35005=VERTEX_POINT('',#183485);
#35006=VERTEX_POINT('',#183487);
#35007=VERTEX_POINT('',#183491);
#35008=VERTEX_POINT('',#183495);
#35009=VERTEX_POINT('',#183497);
#35010=VERTEX_POINT('',#183501);
#35011=VERTEX_POINT('',#183503);
#35012=VERTEX_POINT('',#183731);
#35013=VERTEX_POINT('',#183746);
#43284=EDGE_CURVE('',#34941,#34941,#31337,.T.);
#43285=EDGE_CURVE('',#34941,#34942,#3188,.T.);
#43286=EDGE_CURVE('',#34942,#34943,#31338,.T.);
#43287=EDGE_CURVE('',#34943,#34942,#31339,.T.);
#43288=EDGE_CURVE('',#34944,#34943,#3189,.T.);
#43289=EDGE_CURVE('',#34945,#34946,#3190,.T.);
#43290=EDGE_CURVE('',#34947,#34945,#30274,.F.);
#43291=EDGE_CURVE('',#34948,#34947,#31340,.T.);
#43292=EDGE_CURVE('',#34946,#34948,#30275,.F.);
#43293=EDGE_CURVE('',#34949,#34950,#3191,.T.);
#43294=EDGE_CURVE('',#34945,#34949,#30276,.F.);
#43295=EDGE_CURVE('',#34950,#34946,#30277,.F.);
#43296=EDGE_CURVE('',#34951,#34952,#3192,.T.);
#43297=EDGE_CURVE('',#34949,#34951,#30278,.F.);
#43298=EDGE_CURVE('',#34952,#34950,#30279,.F.);
#43299=EDGE_CURVE('',#34953,#34954,#3193,.T.);
#43300=EDGE_CURVE('',#34948,#34953,#30280,.F.);
#43301=EDGE_CURVE('',#34954,#34948,#31341,.T.);
#43302=EDGE_CURVE('',#34955,#34956,#3194,.T.);
#43303=EDGE_CURVE('',#34957,#34955,#30281,.F.);
#43304=EDGE_CURVE('',#34957,#34958,#31342,.T.);
#43305=EDGE_CURVE('',#34956,#34958,#30282,.F.);
#43306=EDGE_CURVE('',#34959,#34960,#3195,.T.);
#43307=EDGE_CURVE('',#34955,#34959,#30283,.F.);
#43308=EDGE_CURVE('',#34960,#34956,#30284,.F.);
#43309=EDGE_CURVE('',#34961,#34961,#31343,.T.);
#43310=EDGE_CURVE('',#34961,#34962,#3196,.T.);
#43311=EDGE_CURVE('',#34962,#34963,#31344,.T.);
#43312=EDGE_CURVE('',#34963,#34964,#3197,.T.);
#43313=EDGE_CURVE('',#34965,#34964,#31345,.T.);
#43314=EDGE_CURVE('',#34965,#34966,#3198,.T.);
#43315=EDGE_CURVE('',#34966,#34967,#31346,.T.);
#43316=EDGE_CURVE('',#34967,#34968,#3199,.T.);
#43317=EDGE_CURVE('',#34969,#34968,#31347,.T.);
#43318=EDGE_CURVE('',#34969,#34970,#3200,.T.);
#43319=EDGE_CURVE('',#34970,#34962,#31348,.T.);
#43320=EDGE_CURVE('',#34971,#34972,#31349,.T.);
#43321=EDGE_CURVE('',#34971,#34967,#30285,.T.);
#43322=EDGE_CURVE('',#34966,#34972,#1800,.T.);
#43323=EDGE_CURVE('',#34973,#34973,#31350,.T.);
#43324=EDGE_CURVE('',#34973,#34974,#3201,.T.);
#43325=EDGE_CURVE('',#34974,#34974,#31351,.T.);
#43326=EDGE_CURVE('',#34975,#34960,#30286,.F.);
#43327=EDGE_CURVE('',#34975,#34976,#31352,.T.);
#43328=EDGE_CURVE('',#34959,#34976,#30287,.F.);
#43329=EDGE_CURVE('',#34977,#34978,#30288,.F.);
#43330=EDGE_CURVE('',#34977,#34979,#31353,.T.);
#43331=EDGE_CURVE('',#34958,#34979,#31354,.T.);
#43332=EDGE_CURVE('',#34978,#34957,#30289,.F.);
#43333=EDGE_CURVE('',#34978,#34973,#3202,.T.);
#43334=EDGE_CURVE('',#34980,#34981,#31355,.T.);
#43335=EDGE_CURVE('',#34981,#34982,#3203,.T.);
#43336=EDGE_CURVE('',#34982,#34982,#31356,.T.);
#43337=EDGE_CURVE('',#34981,#34980,#31357,.T.);
#43338=EDGE_CURVE('',#34983,#34984,#31358,.T.);
#43339=EDGE_CURVE('',#34984,#34985,#31359,.T.);
#43340=EDGE_CURVE('',#34986,#34985,#3204,.T.);
#43341=EDGE_CURVE('',#34986,#34987,#31360,.T.);
#43342=EDGE_CURVE('',#34987,#34988,#31361,.T.);
#43343=EDGE_CURVE('',#34983,#34988,#3205,.T.);
#43344=EDGE_CURVE('',#34988,#34986,#30290,.F.);
#43345=EDGE_CURVE('',#34987,#34989,#3206,.T.);
#43346=EDGE_CURVE('',#34989,#34989,#31362,.T.);
#43347=EDGE_CURVE('',#34985,#34983,#30291,.F.);
#43348=EDGE_CURVE('',#34984,#34990,#3207,.T.);
#43349=EDGE_CURVE('',#34990,#34990,#31363,.T.);
#43350=EDGE_CURVE('',#34947,#34954,#31364,.T.);
#43351=EDGE_CURVE('',#34991,#34947,#30292,.T.);
#43352=EDGE_CURVE('',#34976,#34991,#30293,.T.);
#43353=EDGE_CURVE('',#34953,#34975,#30294,.F.);
#43354=EDGE_CURVE('',#34980,#34992,#3208,.T.);
#43355=EDGE_CURVE('',#34992,#34992,#31365,.T.);
#43356=EDGE_CURVE('',#34979,#34952,#30295,.F.);
#43357=EDGE_CURVE('',#34951,#34977,#30296,.F.);
#43358=EDGE_CURVE('',#34993,#34993,#31366,.T.);
#43359=EDGE_CURVE('',#34993,#34994,#3209,.T.);
#43360=EDGE_CURVE('',#34994,#34994,#31367,.T.);
#43361=EDGE_CURVE('',#34994,#34995,#31368,.T.);
#43362=EDGE_CURVE('',#34995,#34995,#31369,.T.);
#43363=EDGE_CURVE('',#34995,#34996,#3210,.T.);
#43364=EDGE_CURVE('',#34996,#34996,#31370,.T.);
#43365=EDGE_CURVE('',#34997,#34998,#31371,.T.);
#43366=EDGE_CURVE('',#34998,#34999,#3211,.T.);
#43367=EDGE_CURVE('',#34999,#34999,#31372,.T.);
#43368=EDGE_CURVE('',#34998,#34997,#31373,.T.);
#43369=EDGE_CURVE('',#35000,#35000,#31374,.T.);
#43370=EDGE_CURVE('',#35000,#35001,#3212,.T.);
#43371=EDGE_CURVE('',#35001,#35002,#31375,.T.);
#43372=EDGE_CURVE('',#35002,#35001,#31376,.T.);
#43373=EDGE_CURVE('',#35003,#35003,#31377,.T.);
#43374=EDGE_CURVE('',#35003,#35000,#31378,.T.);
#43375=EDGE_CURVE('',#35004,#35004,#31379,.T.);
#43376=EDGE_CURVE('',#35004,#35002,#31380,.T.);
#43377=EDGE_CURVE('',#34997,#35004,#31381,.T.);
#43378=EDGE_CURVE('',#35005,#35005,#31382,.T.);
#43379=EDGE_CURVE('',#35005,#35006,#3213,.T.);
#43380=EDGE_CURVE('',#35006,#35006,#31383,.T.);
#43381=EDGE_CURVE('',#35006,#35007,#31384,.T.);
#43382=EDGE_CURVE('',#35007,#35007,#31385,.T.);
#43383=EDGE_CURVE('',#35008,#35008,#31386,.T.);
#43384=EDGE_CURVE('',#35008,#35009,#3214,.T.);
#43385=EDGE_CURVE('',#35009,#35009,#31387,.T.);
#43386=EDGE_CURVE('',#35010,#35010,#31388,.T.);
#43387=EDGE_CURVE('',#35010,#35011,#3215,.T.);
#43388=EDGE_CURVE('',#35011,#35011,#31389,.T.);
#43389=EDGE_CURVE('',#34965,#34964,#3216,.T.);
#43390=EDGE_CURVE('',#35012,#34963,#30297,.T.);
#43391=EDGE_CURVE('',#34972,#35012,#3217,.T.);
#43392=EDGE_CURVE('',#34969,#34968,#3218,.T.);
#43393=EDGE_CURVE('',#35013,#34971,#3219,.T.);
#43394=EDGE_CURVE('',#34970,#35013,#1801,.T.);
#43395=EDGE_CURVE('',#35012,#35013,#31390,.T.);
#56903=ORIENTED_EDGE('',*,*,#43284,.T.);
#56904=ORIENTED_EDGE('',*,*,#43285,.T.);
#56905=ORIENTED_EDGE('',*,*,#43286,.T.);
#56906=ORIENTED_EDGE('',*,*,#43287,.T.);
#56907=ORIENTED_EDGE('',*,*,#43285,.F.);
#56908=ORIENTED_EDGE('',*,*,#43288,.T.);
#56909=ORIENTED_EDGE('',*,*,#43286,.F.);
#56910=ORIENTED_EDGE('',*,*,#43287,.F.);
#56911=ORIENTED_EDGE('',*,*,#43288,.F.);
#56912=ORIENTED_EDGE('',*,*,#43284,.F.);
#56913=ORIENTED_EDGE('',*,*,#43289,.F.);
#56914=ORIENTED_EDGE('',*,*,#43290,.F.);
#56915=ORIENTED_EDGE('',*,*,#43291,.F.);
#56916=ORIENTED_EDGE('',*,*,#43292,.F.);
#56917=ORIENTED_EDGE('',*,*,#43293,.F.);
#56918=ORIENTED_EDGE('',*,*,#43294,.F.);
#56919=ORIENTED_EDGE('',*,*,#43289,.T.);
#56920=ORIENTED_EDGE('',*,*,#43295,.F.);
#56921=ORIENTED_EDGE('',*,*,#43296,.F.);
#56922=ORIENTED_EDGE('',*,*,#43297,.F.);
#56923=ORIENTED_EDGE('',*,*,#43293,.T.);
#56924=ORIENTED_EDGE('',*,*,#43298,.F.);
#56925=ORIENTED_EDGE('',*,*,#43299,.F.);
#56926=ORIENTED_EDGE('',*,*,#43300,.F.);
#56927=ORIENTED_EDGE('',*,*,#43301,.F.);
#56928=ORIENTED_EDGE('',*,*,#43302,.F.);
#56929=ORIENTED_EDGE('',*,*,#43303,.F.);
#56930=ORIENTED_EDGE('',*,*,#43304,.T.);
#56931=ORIENTED_EDGE('',*,*,#43305,.F.);
#56932=ORIENTED_EDGE('',*,*,#43306,.F.);
#56933=ORIENTED_EDGE('',*,*,#43307,.F.);
#56934=ORIENTED_EDGE('',*,*,#43302,.T.);
#56935=ORIENTED_EDGE('',*,*,#43308,.F.);
#56936=ORIENTED_EDGE('',*,*,#43309,.T.);
#56937=ORIENTED_EDGE('',*,*,#43310,.T.);
#56938=ORIENTED_EDGE('',*,*,#43311,.T.);
#56939=ORIENTED_EDGE('',*,*,#43312,.T.);
#56940=ORIENTED_EDGE('',*,*,#43313,.F.);
#56941=ORIENTED_EDGE('',*,*,#43314,.T.);
#56942=ORIENTED_EDGE('',*,*,#43315,.T.);
#56943=ORIENTED_EDGE('',*,*,#43316,.T.);
#56944=ORIENTED_EDGE('',*,*,#43317,.F.);
#56945=ORIENTED_EDGE('',*,*,#43318,.T.);
#56946=ORIENTED_EDGE('',*,*,#43319,.T.);
#56947=ORIENTED_EDGE('',*,*,#43310,.F.);
#56948=ORIENTED_EDGE('',*,*,#43320,.F.);
#56949=ORIENTED_EDGE('',*,*,#43321,.T.);
#56950=ORIENTED_EDGE('',*,*,#43315,.F.);
#56951=ORIENTED_EDGE('',*,*,#43322,.T.);
#56952=ORIENTED_EDGE('',*,*,#43323,.F.);
#56953=ORIENTED_EDGE('',*,*,#43324,.T.);
#56954=ORIENTED_EDGE('',*,*,#43325,.T.);
#56955=ORIENTED_EDGE('',*,*,#43324,.F.);
#56956=ORIENTED_EDGE('',*,*,#43306,.T.);
#56957=ORIENTED_EDGE('',*,*,#43326,.F.);
#56958=ORIENTED_EDGE('',*,*,#43327,.T.);
#56959=ORIENTED_EDGE('',*,*,#43328,.F.);
#56960=ORIENTED_EDGE('',*,*,#43329,.F.);
#56961=ORIENTED_EDGE('',*,*,#43330,.T.);
#56962=ORIENTED_EDGE('',*,*,#43331,.F.);
#56963=ORIENTED_EDGE('',*,*,#43304,.F.);
#56964=ORIENTED_EDGE('',*,*,#43332,.F.);
#56965=ORIENTED_EDGE('',*,*,#43333,.T.);
#56966=ORIENTED_EDGE('',*,*,#43323,.T.);
#56967=ORIENTED_EDGE('',*,*,#43333,.F.);
#56968=ORIENTED_EDGE('',*,*,#43334,.T.);
#56969=ORIENTED_EDGE('',*,*,#43335,.T.);
#56970=ORIENTED_EDGE('',*,*,#43336,.T.);
#56971=ORIENTED_EDGE('',*,*,#43335,.F.);
#56972=ORIENTED_EDGE('',*,*,#43337,.T.);
#56973=ORIENTED_EDGE('',*,*,#43338,.T.);
#56974=ORIENTED_EDGE('',*,*,#43339,.T.);
#56975=ORIENTED_EDGE('',*,*,#43340,.F.);
#56976=ORIENTED_EDGE('',*,*,#43341,.T.);
#56977=ORIENTED_EDGE('',*,*,#43342,.T.);
#56978=ORIENTED_EDGE('',*,*,#43343,.F.);
#56979=ORIENTED_EDGE('',*,*,#43341,.F.);
#56980=ORIENTED_EDGE('',*,*,#43344,.F.);
#56981=ORIENTED_EDGE('',*,*,#43342,.F.);
#56982=ORIENTED_EDGE('',*,*,#43345,.T.);
#56983=ORIENTED_EDGE('',*,*,#43346,.F.);
#56984=ORIENTED_EDGE('',*,*,#43345,.F.);
#56985=ORIENTED_EDGE('',*,*,#43338,.F.);
#56986=ORIENTED_EDGE('',*,*,#43347,.F.);
#56987=ORIENTED_EDGE('',*,*,#43339,.F.);
#56988=ORIENTED_EDGE('',*,*,#43348,.T.);
#56989=ORIENTED_EDGE('',*,*,#43349,.F.);
#56990=ORIENTED_EDGE('',*,*,#43348,.F.);
#56991=ORIENTED_EDGE('',*,*,#43299,.T.);
#56992=ORIENTED_EDGE('',*,*,#43350,.F.);
#56993=ORIENTED_EDGE('',*,*,#43351,.F.);
#56994=ORIENTED_EDGE('',*,*,#43352,.F.);
#56995=ORIENTED_EDGE('',*,*,#43327,.F.);
#56996=ORIENTED_EDGE('',*,*,#43353,.F.);
#56997=ORIENTED_EDGE('',*,*,#43334,.F.);
#56998=ORIENTED_EDGE('',*,*,#43354,.T.);
#56999=ORIENTED_EDGE('',*,*,#43355,.F.);
#57000=ORIENTED_EDGE('',*,*,#43354,.F.);
#57001=ORIENTED_EDGE('',*,*,#43337,.F.);
#57002=ORIENTED_EDGE('',*,*,#43296,.T.);
#57003=ORIENTED_EDGE('',*,*,#43356,.F.);
#57004=ORIENTED_EDGE('',*,*,#43330,.F.);
#57005=ORIENTED_EDGE('',*,*,#43357,.F.);
#57006=ORIENTED_EDGE('',*,*,#43358,.F.);
#57007=ORIENTED_EDGE('',*,*,#43359,.T.);
#57008=ORIENTED_EDGE('',*,*,#43360,.T.);
#57009=ORIENTED_EDGE('',*,*,#43359,.F.);
#57010=ORIENTED_EDGE('',*,*,#43360,.F.);
#57011=ORIENTED_EDGE('',*,*,#43361,.T.);
#57012=ORIENTED_EDGE('',*,*,#43362,.T.);
#57013=ORIENTED_EDGE('',*,*,#43361,.F.);
#57014=ORIENTED_EDGE('',*,*,#43362,.F.);
#57015=ORIENTED_EDGE('',*,*,#43363,.T.);
#57016=ORIENTED_EDGE('',*,*,#43364,.T.);
#57017=ORIENTED_EDGE('',*,*,#43363,.F.);
#57018=ORIENTED_EDGE('',*,*,#43365,.T.);
#57019=ORIENTED_EDGE('',*,*,#43366,.T.);
#57020=ORIENTED_EDGE('',*,*,#43367,.T.);
#57021=ORIENTED_EDGE('',*,*,#43366,.F.);
#57022=ORIENTED_EDGE('',*,*,#43368,.T.);
#57023=ORIENTED_EDGE('',*,*,#43369,.T.);
#57024=ORIENTED_EDGE('',*,*,#43370,.T.);
#57025=ORIENTED_EDGE('',*,*,#43371,.T.);
#57026=ORIENTED_EDGE('',*,*,#43372,.T.);
#57027=ORIENTED_EDGE('',*,*,#43370,.F.);
#57028=ORIENTED_EDGE('',*,*,#43373,.F.);
#57029=ORIENTED_EDGE('',*,*,#43374,.T.);
#57030=ORIENTED_EDGE('',*,*,#43369,.F.);
#57031=ORIENTED_EDGE('',*,*,#43374,.F.);
#57032=ORIENTED_EDGE('',*,*,#43375,.F.);
#57033=ORIENTED_EDGE('',*,*,#43376,.T.);
#57034=ORIENTED_EDGE('',*,*,#43371,.F.);
#57035=ORIENTED_EDGE('',*,*,#43372,.F.);
#57036=ORIENTED_EDGE('',*,*,#43376,.F.);
#57037=ORIENTED_EDGE('',*,*,#43365,.F.);
#57038=ORIENTED_EDGE('',*,*,#43377,.T.);
#57039=ORIENTED_EDGE('',*,*,#43375,.T.);
#57040=ORIENTED_EDGE('',*,*,#43377,.F.);
#57041=ORIENTED_EDGE('',*,*,#43368,.F.);
#57042=ORIENTED_EDGE('',*,*,#43378,.F.);
#57043=ORIENTED_EDGE('',*,*,#43379,.T.);
#57044=ORIENTED_EDGE('',*,*,#43380,.T.);
#57045=ORIENTED_EDGE('',*,*,#43379,.F.);
#57046=ORIENTED_EDGE('',*,*,#43380,.F.);
#57047=ORIENTED_EDGE('',*,*,#43381,.T.);
#57048=ORIENTED_EDGE('',*,*,#43382,.F.);
#57049=ORIENTED_EDGE('',*,*,#43381,.F.);
#57050=ORIENTED_EDGE('',*,*,#43383,.F.);
#57051=ORIENTED_EDGE('',*,*,#43384,.T.);
#57052=ORIENTED_EDGE('',*,*,#43385,.T.);
#57053=ORIENTED_EDGE('',*,*,#43384,.F.);
#57054=ORIENTED_EDGE('',*,*,#43386,.T.);
#57055=ORIENTED_EDGE('',*,*,#43387,.T.);
#57056=ORIENTED_EDGE('',*,*,#43388,.T.);
#57057=ORIENTED_EDGE('',*,*,#43387,.F.);
#57058=ORIENTED_EDGE('',*,*,#43347,.T.);
#57059=ORIENTED_EDGE('',*,*,#43343,.T.);
#57060=ORIENTED_EDGE('',*,*,#43344,.T.);
#57061=ORIENTED_EDGE('',*,*,#43340,.T.);
#57062=ORIENTED_EDGE('',*,*,#43383,.T.);
#57063=ORIENTED_EDGE('',*,*,#43386,.F.);
#57064=ORIENTED_EDGE('',*,*,#43382,.T.);
#57065=ORIENTED_EDGE('',*,*,#43385,.F.);
#57066=ORIENTED_EDGE('',*,*,#43373,.T.);
#57067=ORIENTED_EDGE('',*,*,#43367,.F.);
#57068=ORIENTED_EDGE('',*,*,#43378,.T.);
#57069=ORIENTED_EDGE('',*,*,#43364,.F.);
#57070=ORIENTED_EDGE('',*,*,#43358,.T.);
#57071=ORIENTED_EDGE('',*,*,#43388,.F.);
#57072=ORIENTED_EDGE('',*,*,#43329,.T.);
#57073=ORIENTED_EDGE('',*,*,#43332,.T.);
#57074=ORIENTED_EDGE('',*,*,#43303,.T.);
#57075=ORIENTED_EDGE('',*,*,#43307,.T.);
#57076=ORIENTED_EDGE('',*,*,#43328,.T.);
#57077=ORIENTED_EDGE('',*,*,#43352,.T.);
#57078=ORIENTED_EDGE('',*,*,#43351,.T.);
#57079=ORIENTED_EDGE('',*,*,#43290,.T.);
#57080=ORIENTED_EDGE('',*,*,#43294,.T.);
#57081=ORIENTED_EDGE('',*,*,#43297,.T.);
#57082=ORIENTED_EDGE('',*,*,#43357,.T.);
#57083=ORIENTED_EDGE('',*,*,#43331,.T.);
#57084=ORIENTED_EDGE('',*,*,#43356,.T.);
#57085=ORIENTED_EDGE('',*,*,#43298,.T.);
#57086=ORIENTED_EDGE('',*,*,#43295,.T.);
#57087=ORIENTED_EDGE('',*,*,#43292,.T.);
#57088=ORIENTED_EDGE('',*,*,#43300,.T.);
#57089=ORIENTED_EDGE('',*,*,#43353,.T.);
#57090=ORIENTED_EDGE('',*,*,#43326,.T.);
#57091=ORIENTED_EDGE('',*,*,#43308,.T.);
#57092=ORIENTED_EDGE('',*,*,#43305,.T.);
#57093=ORIENTED_EDGE('',*,*,#43313,.T.);
#57094=ORIENTED_EDGE('',*,*,#43389,.F.);
#57095=ORIENTED_EDGE('',*,*,#43389,.T.);
#57096=ORIENTED_EDGE('',*,*,#43312,.F.);
#57097=ORIENTED_EDGE('',*,*,#43390,.F.);
#57098=ORIENTED_EDGE('',*,*,#43391,.F.);
#57099=ORIENTED_EDGE('',*,*,#43322,.F.);
#57100=ORIENTED_EDGE('',*,*,#43314,.F.);
#57101=ORIENTED_EDGE('',*,*,#43317,.T.);
#57102=ORIENTED_EDGE('',*,*,#43392,.F.);
#57103=ORIENTED_EDGE('',*,*,#43392,.T.);
#57104=ORIENTED_EDGE('',*,*,#43316,.F.);
#57105=ORIENTED_EDGE('',*,*,#43321,.F.);
#57106=ORIENTED_EDGE('',*,*,#43393,.F.);
#57107=ORIENTED_EDGE('',*,*,#43394,.F.);
#57108=ORIENTED_EDGE('',*,*,#43318,.F.);
#57109=ORIENTED_EDGE('',*,*,#43336,.F.);
#57110=ORIENTED_EDGE('',*,*,#43349,.T.);
#57111=ORIENTED_EDGE('',*,*,#43291,.T.);
#57112=ORIENTED_EDGE('',*,*,#43350,.T.);
#57113=ORIENTED_EDGE('',*,*,#43301,.T.);
#57114=ORIENTED_EDGE('',*,*,#43355,.T.);
#57115=ORIENTED_EDGE('',*,*,#43309,.F.);
#57116=ORIENTED_EDGE('',*,*,#43325,.F.);
#57117=ORIENTED_EDGE('',*,*,#43395,.F.);
#57118=ORIENTED_EDGE('',*,*,#43390,.T.);
#57119=ORIENTED_EDGE('',*,*,#43311,.F.);
#57120=ORIENTED_EDGE('',*,*,#43319,.F.);
#57121=ORIENTED_EDGE('',*,*,#43394,.T.);
#57122=ORIENTED_EDGE('',*,*,#43320,.T.);
#57123=ORIENTED_EDGE('',*,*,#43391,.T.);
#57124=ORIENTED_EDGE('',*,*,#43395,.T.);
#57125=ORIENTED_EDGE('',*,*,#43393,.T.);
#57126=ORIENTED_EDGE('',*,*,#43346,.T.);
#76221=ADVANCED_FACE('',(#20791),#2254,.F.);
#76222=ADVANCED_FACE('',(#20792),#1947,.F.);
#76223=ADVANCED_FACE('',(#20793),#17003,.T.);
#76224=ADVANCED_FACE('',(#20794),#2255,.T.);
#76225=ADVANCED_FACE('',(#20795),#2256,.T.);
#76226=ADVANCED_FACE('',(#20796),#2257,.T.);
#76227=ADVANCED_FACE('',(#20797),#1948,.T.);
#76228=ADVANCED_FACE('',(#20798),#2258,.T.);
#76229=ADVANCED_FACE('',(#20799),#2259,.T.);
#76230=ADVANCED_FACE('',(#20800),#2260,.T.);
#76231=ADVANCED_FACE('',(#20801),#1949,.T.);
#76232=ADVANCED_FACE('',(#20802),#2261,.T.);
#76233=ADVANCED_FACE('',(#20803),#2262,.T.);
#76234=ADVANCED_FACE('',(#20804),#1950,.T.);
#76235=ADVANCED_FACE('',(#20805),#2263,.F.);
#76236=ADVANCED_FACE('',(#20806),#2264,.F.);
#76237=ADVANCED_FACE('',(#20807),#1951,.F.);
#76238=ADVANCED_FACE('',(#20808),#1952,.F.);
#76239=ADVANCED_FACE('',(#20809),#1953,.T.);
#76240=ADVANCED_FACE('',(#20810),#1954,.F.);
#76241=ADVANCED_FACE('',(#20811),#2265,.T.);
#76242=ADVANCED_FACE('',(#20812),#2266,.T.);
#76243=ADVANCED_FACE('',(#20813),#1898,.T.);
#76244=ADVANCED_FACE('',(#20814),#2267,.T.);
#76245=ADVANCED_FACE('',(#20815),#2268,.T.);
#76246=ADVANCED_FACE('',(#20816),#2269,.T.);
#76247=ADVANCED_FACE('',(#20817),#1899,.T.);
#76248=ADVANCED_FACE('',(#20818),#1900,.T.);
#76249=ADVANCED_FACE('',(#20819),#1901,.F.);
#76250=ADVANCED_FACE('',(#20820),#2270,.F.);
#76251=ADVANCED_FACE('',(#20821),#1902,.F.);
#76252=ADVANCED_FACE('',(#20822),#2271,.T.);
#76253=ADVANCED_FACE('',(#20823,#305),#2272,.T.);
#76254=ADVANCED_FACE('',(#20824,#306),#17004,.T.);
#76255=ADVANCED_FACE('',(#20825,#307),#17005,.F.);
#76256=ADVANCED_FACE('',(#20826),#17006,.T.);
#76257=ADVANCED_FACE('',(#20827,#308),#17007,.T.);
#76258=ADVANCED_FACE('',(#20828),#17008,.T.);
#76259=ADVANCED_FACE('',(#20829,#309),#17009,.T.);
#76260=ADVANCED_FACE('',(#20830),#199,.F.);
#76261=ADVANCED_FACE('',(#20831),#200,.F.);
#76262=ADVANCED_FACE('',(#20832),#17010,.F.);
#76263=ADVANCED_FACE('',(#20833),#17011,.T.);
#76264=ADVANCED_FACE('',(#20834),#17012,.F.);
#76265=ADVANCED_FACE('',(#20835),#17013,.T.);
#76266=ADVANCED_FACE('',(#20836,#310),#17014,.F.);
#76267=ADVANCED_FACE('',(#20837,#311),#17015,.T.);
#76268=ADVANCED_FACE('',(#20838,#312),#17016,.T.);
#76269=ADVANCED_FACE('',(#20839),#1955,.T.);
#76270=ADVANCED_FACE('',(#20840,#313),#17017,.T.);
#79330=CLOSED_SHELL('',(#76221,#76222,#76223));
#79331=CLOSED_SHELL('',(#76224,#76225,#76226,#76227,#76228,#76229,#76230,
#76231,#76232,#76233,#76234,#76235,#76236,#76237,#76238,#76239,#76240,#76241,
#76242,#76243,#76244,#76245,#76246,#76247,#76248,#76249,#76250,#76251,#76252,
#76253,#76254,#76255,#76256,#76257,#76258,#76259,#76260,#76261,#76262,#76263,
#76264,#76265,#76266,#76267,#76268,#76269,#76270));
#79337=BREP_WITH_VOIDS('Body1',#79331,(#1979));
#80848=AXIS2_PLACEMENT_3D('',#181110,#89383,#89384);
#80849=AXIS2_PLACEMENT_3D('',#181111,#89385,#89386);
#80850=AXIS2_PLACEMENT_3D('',#181113,#89387,#89388);
#80851=AXIS2_PLACEMENT_3D('',#181117,#89390,#89391);
#80852=AXIS2_PLACEMENT_3D('',#181118,#89392,#89393);
#80853=AXIS2_PLACEMENT_3D('',#181119,#89394,#89395);
#80854=AXIS2_PLACEMENT_3D('',#181122,#89397,#89398);
#80855=AXIS2_PLACEMENT_3D('',#181123,#89399,#89400);
#80856=AXIS2_PLACEMENT_3D('',#181239,#89402,#89403);
#80857=AXIS2_PLACEMENT_3D('',#181316,#89404,#89405);
#80858=AXIS2_PLACEMENT_3D('',#181680,#89407,#89408);
#80859=AXIS2_PLACEMENT_3D('',#182042,#89410,#89411);
#80860=AXIS2_PLACEMENT_3D('',#182064,#89413,#89414);
#80861=AXIS2_PLACEMENT_3D('',#182065,#89415,#89416);
#80862=AXIS2_PLACEMENT_3D('',#182149,#89418,#89419);
#80863=AXIS2_PLACEMENT_3D('',#182206,#89420,#89421);
#80864=AXIS2_PLACEMENT_3D('',#182588,#89423,#89424);
#80865=AXIS2_PLACEMENT_3D('',#182590,#89425,#89426);
#80866=AXIS2_PLACEMENT_3D('',#182594,#89428,#89429);
#80867=AXIS2_PLACEMENT_3D('',#182598,#89431,#89432);
#80868=AXIS2_PLACEMENT_3D('',#182602,#89434,#89435);
#80869=AXIS2_PLACEMENT_3D('',#182606,#89437,#89438);
#80870=AXIS2_PLACEMENT_3D('',#182609,#89440,#89441);
#80871=AXIS2_PLACEMENT_3D('',#182610,#89442,#89443);
#80872=AXIS2_PLACEMENT_3D('',#182613,#89444,#89445);
#80873=AXIS2_PLACEMENT_3D('',#182627,#89446,#89447);
#80874=AXIS2_PLACEMENT_3D('',#182629,#89448,#89449);
#80875=AXIS2_PLACEMENT_3D('',#182632,#89451,#89452);
#80876=AXIS2_PLACEMENT_3D('',#182633,#89453,#89454);
#80877=AXIS2_PLACEMENT_3D('',#182812,#89455,#89456);
#80878=AXIS2_PLACEMENT_3D('',#182973,#89457,#89458);
#80879=AXIS2_PLACEMENT_3D('',#182983,#89459,#89460);
#80880=AXIS2_PLACEMENT_3D('',#182984,#89461,#89462);
#80881=AXIS2_PLACEMENT_3D('',#183012,#89464,#89465);
#80882=AXIS2_PLACEMENT_3D('',#183015,#89466,#89467);
#80883=AXIS2_PLACEMENT_3D('',#183018,#89469,#89470);
#80884=AXIS2_PLACEMENT_3D('',#183019,#89471,#89472);
#80885=AXIS2_PLACEMENT_3D('',#183020,#89473,#89474);
#80886=AXIS2_PLACEMENT_3D('',#183023,#89475,#89476);
#80887=AXIS2_PLACEMENT_3D('',#183025,#89477,#89478);
#80888=AXIS2_PLACEMENT_3D('',#183029,#89480,#89481);
#80889=AXIS2_PLACEMENT_3D('',#183031,#89482,#89483);
#80890=AXIS2_PLACEMENT_3D('',#183033,#89485,#89486);
#80891=AXIS2_PLACEMENT_3D('',#183044,#89488,#89489);
#80892=AXIS2_PLACEMENT_3D('',#183045,#89490,#89491);
#80893=AXIS2_PLACEMENT_3D('',#183055,#89493,#89494);
#80894=AXIS2_PLACEMENT_3D('',#183056,#89495,#89496);
#80895=AXIS2_PLACEMENT_3D('',#183057,#89497,#89498);
#80896=AXIS2_PLACEMENT_3D('',#183185,#89499,#89500);
#80897=AXIS2_PLACEMENT_3D('',#183188,#89502,#89503);
#80898=AXIS2_PLACEMENT_3D('',#183189,#89504,#89505);
#80899=AXIS2_PLACEMENT_3D('',#183444,#89506,#89507);
#80900=AXIS2_PLACEMENT_3D('',#183446,#89508,#89509);
#80901=AXIS2_PLACEMENT_3D('',#183449,#89511,#89512);
#80902=AXIS2_PLACEMENT_3D('',#183450,#89513,#89514);
#80903=AXIS2_PLACEMENT_3D('',#183452,#89515,#89516);
#80904=AXIS2_PLACEMENT_3D('',#183453,#89517,#89518);
#80905=AXIS2_PLACEMENT_3D('',#183454,#89519,#89520);
#80906=AXIS2_PLACEMENT_3D('',#183457,#89522,#89523);
#80907=AXIS2_PLACEMENT_3D('',#183458,#89524,#89525);
#80908=AXIS2_PLACEMENT_3D('',#183461,#89526,#89527);
#80909=AXIS2_PLACEMENT_3D('',#183464,#89529,#89530);
#80910=AXIS2_PLACEMENT_3D('',#183465,#89531,#89532);
#80911=AXIS2_PLACEMENT_3D('',#183466,#89533,#89534);
#80912=AXIS2_PLACEMENT_3D('',#183468,#89535,#89536);
#80913=AXIS2_PLACEMENT_3D('',#183472,#89538,#89539);
#80914=AXIS2_PLACEMENT_3D('',#183473,#89540,#89541);
#80915=AXIS2_PLACEMENT_3D('',#183474,#89542,#89543);
#80916=AXIS2_PLACEMENT_3D('',#183476,#89544,#89545);
#80917=AXIS2_PLACEMENT_3D('',#183477,#89546,#89547);
#80918=AXIS2_PLACEMENT_3D('',#183478,#89548,#89549);
#80919=AXIS2_PLACEMENT_3D('',#183480,#89550,#89551);
#80920=AXIS2_PLACEMENT_3D('',#183481,#89552,#89553);
#80921=AXIS2_PLACEMENT_3D('',#183482,#89554,#89555);
#80922=AXIS2_PLACEMENT_3D('',#183483,#89556,#89557);
#80923=AXIS2_PLACEMENT_3D('',#183484,#89558,#89559);
#80924=AXIS2_PLACEMENT_3D('',#183486,#89560,#89561);
#80925=AXIS2_PLACEMENT_3D('',#183489,#89563,#89564);
#80926=AXIS2_PLACEMENT_3D('',#183490,#89565,#89566);
#80927=AXIS2_PLACEMENT_3D('',#183492,#89567,#89568);
#80928=AXIS2_PLACEMENT_3D('',#183493,#89569,#89570);
#80929=AXIS2_PLACEMENT_3D('',#183494,#89571,#89572);
#80930=AXIS2_PLACEMENT_3D('',#183496,#89573,#89574);
#80931=AXIS2_PLACEMENT_3D('',#183499,#89576,#89577);
#80932=AXIS2_PLACEMENT_3D('',#183500,#89578,#89579);
#80933=AXIS2_PLACEMENT_3D('',#183502,#89580,#89581);
#80934=AXIS2_PLACEMENT_3D('',#183505,#89583,#89584);
#80935=AXIS2_PLACEMENT_3D('',#183506,#89585,#89586);
#80936=AXIS2_PLACEMENT_3D('',#183507,#89587,#89588);
#80937=AXIS2_PLACEMENT_3D('',#183508,#89589,#89590);
#80938=AXIS2_PLACEMENT_3D('',#183509,#89591,#89592);
#80939=AXIS2_PLACEMENT_3D('',#183510,#89593,#89594);
#80940=AXIS2_PLACEMENT_3D('',#183511,#89595,#89596);
#80941=AXIS2_PLACEMENT_3D('',#183728,#89597,#89598);
#80942=AXIS2_PLACEMENT_3D('',#183730,#89600,#89601);
#80943=AXIS2_PLACEMENT_3D('',#183743,#89603,#89604);
#80944=AXIS2_PLACEMENT_3D('',#183745,#89606,#89607);
#80945=AXIS2_PLACEMENT_3D('',#183751,#89609,#89610);
#80946=AXIS2_PLACEMENT_3D('',#183752,#89611,#89612);
#80947=AXIS2_PLACEMENT_3D('',#183753,#89613,#89614);
#80948=AXIS2_PLACEMENT_3D('',#183754,#89615,#89616);
#80949=AXIS2_PLACEMENT_3D('',#183755,#89617,#89618);
#80950=AXIS2_PLACEMENT_3D('',#183756,#89619,#89620);
#89383=DIRECTION('axis',(0.,0.,1.));
#89384=DIRECTION('refdir',(1.,0.,0.));
#89385=DIRECTION('center_axis',(0.173648177666905,0.,0.984807753012213));
#89386=DIRECTION('ref_axis',(0.984807753012213,0.,-0.173648177666905));
#89387=DIRECTION('center_axis',(-0.173648177666884,0.,-0.984807753012216));
#89388=DIRECTION('ref_axis',(0.984807753012216,0.,-0.173648177666884));
#89389=DIRECTION('',(0.173648177666905,0.,0.984807753012213));
#89390=DIRECTION('center_axis',(0.173648177666905,0.,0.984807753012213));
#89391=DIRECTION('ref_axis',(0.984807753012213,0.,-0.173648177666905));
#89392=DIRECTION('center_axis',(0.173648177666905,0.,0.984807753012213));
#89393=DIRECTION('ref_axis',(0.984807753012213,0.,-0.173648177666905));
#89394=DIRECTION('center_axis',(-0.173648177666902,0.,-0.984807753012213));
#89395=DIRECTION('ref_axis',(-0.984807753012213,0.,0.173648177666902));
#89396=DIRECTION('',(0.754709579450836,-1.04972719039646E-16,-0.656059029878518));
#89397=DIRECTION('center_axis',(0.173648177666884,0.,0.984807753012216));
#89398=DIRECTION('ref_axis',(0.984807753012216,0.,-0.173648177666884));
#89399=DIRECTION('center_axis',(0.173648177666902,6.42277782841E-16,0.984807753012213));
#89400=DIRECTION('ref_axis',(0.171010071662809,-0.984807753012213,-0.0301536896070356));
#89401=DIRECTION('',(-0.173648177666902,-6.42277782841E-16,-0.984807753012213));
#89402=DIRECTION('center_axis',(-0.173648177666902,-6.42277782841E-16,-0.984807753012213));
#89403=DIRECTION('ref_axis',(-0.171010071662809,0.984807753012213,0.0301536896070356));
#89404=DIRECTION('center_axis',(0.173648177666902,6.42277782841E-16,0.984807753012213));
#89405=DIRECTION('ref_axis',(0.171010071662809,-0.984807753012213,-0.0301536896070356));
#89406=DIRECTION('',(-0.173648177666902,-6.42277782841E-16,-0.984807753012213));
#89407=DIRECTION('center_axis',(0.173648177666902,6.42277782841E-16,0.984807753012213));
#89408=DIRECTION('ref_axis',(0.171010071662809,-0.984807753012213,-0.0301536896070356));
#89409=DIRECTION('',(-0.173648177666902,-6.42277782841E-16,-0.984807753012213));
#89410=DIRECTION('center_axis',(0.173648177666902,-1.13774921531834E-16,
0.984807753012213));
#89411=DIRECTION('ref_axis',(0.171010071662809,-0.984807753012213,-0.0301536896070363));
#89412=DIRECTION('',(-0.00186542286370051,-0.696364239695072,-0.717686119324768));
#89413=DIRECTION('center_axis',(-0.173648177666902,-6.42277782841E-16,-0.984807753012213));
#89414=DIRECTION('ref_axis',(-0.171010071662809,0.984807753012213,0.0301536896070356));
#89415=DIRECTION('center_axis',(-0.173648177666902,2.83723661848651E-16,
-0.984807753012213));
#89416=DIRECTION('ref_axis',(-0.171010071662807,0.984807753012213,0.0301536896070362));
#89417=DIRECTION('',(0.173648177666902,-2.83723661848651E-16,0.984807753012213));
#89418=DIRECTION('center_axis',(-0.173648177666902,2.83723661848651E-16,
-0.984807753012213));
#89419=DIRECTION('ref_axis',(0.171010071662807,-0.984807753012213,-0.0301536896070362));
#89420=DIRECTION('center_axis',(-0.173648177666902,2.83723661848651E-16,
-0.984807753012213));
#89421=DIRECTION('ref_axis',(-0.171010071662807,0.984807753012213,0.0301536896070362));
#89422=DIRECTION('',(0.173648177666902,-2.83723661848651E-16,0.984807753012213));
#89423=DIRECTION('center_axis',(-0.173648177666902,-8.51926239304202E-16,
-0.984807753012213));
#89424=DIRECTION('ref_axis',(-0.171010071662808,0.984807753012213,0.0301536896070352));
#89425=DIRECTION('center_axis',(0.173648177666902,8.51926239304202E-16,
0.984807753012213));
#89426=DIRECTION('ref_axis',(0.171010071662808,-0.984807753012213,-0.0301536896070352));
#89427=DIRECTION('',(0.173648177666902,8.51926239304202E-16,0.984807753012213));
#89428=DIRECTION('center_axis',(-0.173648177666902,-8.51926239304202E-16,
-0.984807753012213));
#89429=DIRECTION('ref_axis',(0.171010071662808,-0.984807753012213,-0.0301536896070352));
#89430=DIRECTION('',(-0.173648177666902,0.,-0.984807753012213));
#89431=DIRECTION('center_axis',(0.173648177666902,8.51926239304202E-16,
0.984807753012213));
#89432=DIRECTION('ref_axis',(-0.171010071662808,0.984807753012213,0.0301536896070352));
#89433=DIRECTION('',(0.173648177666902,0.,0.984807753012213));
#89434=DIRECTION('center_axis',(-0.173648177666902,-8.51926239304202E-16,
-0.984807753012213));
#89435=DIRECTION('ref_axis',(0.171010071662808,-0.984807753012213,-0.0301536896070352));
#89436=DIRECTION('',(-0.173648177666902,0.,-0.984807753012213));
#89437=DIRECTION('center_axis',(0.173648177666902,8.51926239304202E-16,
0.984807753012213));
#89438=DIRECTION('ref_axis',(-0.171010071662808,0.984807753012213,0.0301536896070352));
#89439=DIRECTION('',(0.173648177666902,0.,0.984807753012213));
#89440=DIRECTION('center_axis',(-0.173648177666902,-8.51926239304202E-16,
-0.984807753012213));
#89441=DIRECTION('ref_axis',(0.171010071662808,-0.984807753012213,-0.0301536896070352));
#89442=DIRECTION('center_axis',(-0.173648177666902,2.26576127474522E-17,
-0.984807753012213));
#89443=DIRECTION('ref_axis',(-0.171010071662808,0.984807753012213,0.0301536896070361));
#89444=DIRECTION('center_axis',(0.173648177666902,-7.67302066723185E-16,
0.984807753012213));
#89445=DIRECTION('ref_axis',(0.171010071662807,-0.984807753012213,-0.0301536896070368));
#89446=DIRECTION('center_axis',(-0.173648177666902,4.06830024443141E-16,
-0.984807753012213));
#89447=DIRECTION('ref_axis',(-0.171010071662808,0.984807753012213,0.0301536896070366));
#89448=DIRECTION('center_axis',(-0.173648177666902,4.06830024443141E-16,
-0.984807753012213));
#89449=DIRECTION('ref_axis',(-0.171010071662808,0.984807753012213,0.0301536896070366));
#89450=DIRECTION('',(0.173648177666902,-4.06830024443141E-16,0.984807753012213));
#89451=DIRECTION('center_axis',(-0.173648177666902,4.06830024443141E-16,
-0.984807753012213));
#89452=DIRECTION('ref_axis',(-0.171010071662808,0.984807753012213,0.0301536896070366));
#89453=DIRECTION('center_axis',(-0.173648177666902,2.83723661848651E-16,
-0.984807753012213));
#89454=DIRECTION('ref_axis',(-0.171010071662807,0.984807753012213,0.0301536896070362));
#89455=DIRECTION('center_axis',(0.173648177666902,-2.83723661848651E-16,
0.984807753012213));
#89456=DIRECTION('ref_axis',(-0.171010071662807,0.984807753012213,0.0301536896070362));
#89457=DIRECTION('center_axis',(-0.173648177666902,1.8503717077086E-17,
-0.984807753012213));
#89458=DIRECTION('ref_axis',(-0.171010071662807,0.984807753012213,0.0301536896070359));
#89459=DIRECTION('center_axis',(0.173648177666902,6.42277782841E-16,0.984807753012213));
#89460=DIRECTION('ref_axis',(-0.171010071662809,0.984807753012213,0.0301536896070356));
#89461=DIRECTION('center_axis',(-0.605579649361399,-0.190525192352794,-0.772640562848117));
#89462=DIRECTION('ref_axis',(0.381374075544339,-0.921640193904515,-0.0716461267784125));
#89463=DIRECTION('',(-0.0612749772472734,0.852868531363239,0.518517738726129));
#89464=DIRECTION('center_axis',(0.173648177666902,-1.04370139711662E-15,
0.984807753012213));
#89465=DIRECTION('ref_axis',(0.171010071662806,-0.984807753012213,-0.0301536896070368));
#89466=DIRECTION('center_axis',(-0.173648177666902,1.04370139711662E-15,
-0.984807753012213));
#89467=DIRECTION('ref_axis',(-0.171010071662806,0.984807753012213,0.0301536896070368));
#89468=DIRECTION('',(0.173648177666902,-1.04370139711662E-15,0.984807753012213));
#89469=DIRECTION('center_axis',(0.173648177666902,-1.04370139711662E-15,
0.984807753012213));
#89470=DIRECTION('ref_axis',(0.171010071662806,-0.984807753012213,-0.0301536896070368));
#89471=DIRECTION('center_axis',(-0.173648177666902,1.04370139711662E-15,
-0.984807753012213));
#89472=DIRECTION('ref_axis',(-0.171010071662806,0.984807753012213,0.0301536896070368));
#89473=DIRECTION('center_axis',(0.173648177666902,1.22504424478055E-15,
0.984807753012213));
#89474=DIRECTION('ref_axis',(-0.984807753012213,6.95411525205428E-14,0.173648177666902));
#89475=DIRECTION('center_axis',(-0.173648177666902,-1.22504424478055E-15,
-0.984807753012213));
#89476=DIRECTION('ref_axis',(0.171010071662809,-0.984807753012213,-0.0301536896070351));
#89477=DIRECTION('center_axis',(-0.173648177666902,-1.22504424478055E-15,
-0.984807753012213));
#89478=DIRECTION('ref_axis',(0.171010071662809,-0.984807753012213,-0.0301536896070351));
#89479=DIRECTION('',(-0.173648177666902,-1.22504424478055E-15,-0.984807753012213));
#89480=DIRECTION('center_axis',(0.173648177666902,1.22504424478055E-15,
0.984807753012213));
#89481=DIRECTION('ref_axis',(0.171010071662809,-0.984807753012213,-0.0301536896070351));
#89482=DIRECTION('center_axis',(0.173648177666902,1.22504424478055E-15,
0.984807753012213));
#89483=DIRECTION('ref_axis',(0.171010071662809,-0.984807753012213,-0.0301536896070351));
#89484=DIRECTION('',(0.173648177666902,1.22504424478055E-15,0.984807753012213));
#89485=DIRECTION('center_axis',(0.173648177666902,-1.7073787383701E-17,
0.984807753012213));
#89486=DIRECTION('ref_axis',(0.171010071662809,-0.984807753012213,-0.0301536896070363));
#89487=DIRECTION('',(0.00186542286370016,0.696364239695072,0.717686119324768));
#89488=DIRECTION('center_axis',(-0.173648177666902,5.60929665760627E-16,
-0.984807753012213));
#89489=DIRECTION('ref_axis',(0.171010071662806,-0.984807753012213,-0.0301536896070362));
#89490=DIRECTION('center_axis',(-0.173648177666902,1.79020106093818E-17,
-0.984807753012213));
#89491=DIRECTION('ref_axis',(-0.17101007166281,0.984807753012213,0.0301536896070365));
#89492=DIRECTION('',(-0.00186542286369971,-0.696364239695071,-0.717686119324768));
#89493=DIRECTION('center_axis',(0.173648177666902,-5.60929665760627E-16,
0.984807753012213));
#89494=DIRECTION('ref_axis',(0.171010071662806,-0.984807753012213,-0.0301536896070362));
#89495=DIRECTION('center_axis',(0.173648177666902,-1.13774921531834E-16,
0.984807753012213));
#89496=DIRECTION('ref_axis',(0.171010071662809,-0.984807753012213,-0.0301536896070363));
#89497=DIRECTION('center_axis',(-0.173648177666902,-6.42277782841E-16,-0.984807753012213));
#89498=DIRECTION('ref_axis',(-0.171010071662809,0.984807753012213,0.0301536896070356));
#89499=DIRECTION('center_axis',(-0.173648177666902,-8.32320468273753E-17,
-0.984807753012213));
#89500=DIRECTION('ref_axis',(-0.171010071662807,0.984807753012213,0.0301536896070358));
#89501=DIRECTION('',(-0.00186542286370196,-0.696364239695072,-0.717686119324767));
#89502=DIRECTION('center_axis',(0.173648177666903,-1.55366487411101E-15,
0.984807753012213));
#89503=DIRECTION('ref_axis',(-0.171010071662807,0.984807753012213,0.0301536896070375));
#89504=DIRECTION('center_axis',(0.173648177666902,6.42277782841E-16,0.984807753012213));
#89505=DIRECTION('ref_axis',(0.171010071662809,-0.984807753012213,-0.0301536896070356));
#89506=DIRECTION('center_axis',(0.173648177666884,0.,0.984807753012216));
#89507=DIRECTION('ref_axis',(0.984807753012216,0.,-0.173648177666884));
#89508=DIRECTION('center_axis',(0.173648177666884,0.,0.984807753012216));
#89509=DIRECTION('ref_axis',(0.984807753012216,0.,-0.173648177666884));
#89510=DIRECTION('',(-0.173648177666884,0.,-0.984807753012216));
#89511=DIRECTION('center_axis',(0.173648177666884,0.,0.984807753012216));
#89512=DIRECTION('ref_axis',(0.984807753012216,0.,-0.173648177666884));
#89513=DIRECTION('center_axis',(0.173648177666884,0.,0.984807753012216));
#89514=DIRECTION('ref_axis',(0.984807753012216,0.,-0.173648177666883));
#89515=DIRECTION('center_axis',(1.20604166250191E-16,-1.,-2.1265768495752E-17));
#89516=DIRECTION('ref_axis',(-0.984807753012216,-1.22464679914735E-16,0.173648177666884));
#89517=DIRECTION('center_axis',(0.173648177666884,0.,0.984807753012216));
#89518=DIRECTION('ref_axis',(0.984807753012216,0.,-0.173648177666884));
#89519=DIRECTION('center_axis',(0.173648177666884,0.,0.984807753012216));
#89520=DIRECTION('ref_axis',(0.984807753012216,0.,-0.173648177666884));
#89521=DIRECTION('',(-0.173648177666884,0.,-0.984807753012216));
#89522=DIRECTION('center_axis',(0.173648177666884,0.,0.984807753012216));
#89523=DIRECTION('ref_axis',(0.984807753012216,0.,-0.173648177666884));
#89524=DIRECTION('center_axis',(0.173648177666903,0.,0.984807753012213));
#89525=DIRECTION('ref_axis',(0.984807753012213,0.,-0.173648177666903));
#89526=DIRECTION('center_axis',(-0.173648177666903,0.,-0.984807753012213));
#89527=DIRECTION('ref_axis',(-0.984807753012213,0.,0.173648177666903));
#89528=DIRECTION('',(-0.173648177666903,0.,-0.984807753012213));
#89529=DIRECTION('center_axis',(0.173648177666903,0.,0.984807753012213));
#89530=DIRECTION('ref_axis',(0.984807753012213,0.,-0.173648177666903));
#89531=DIRECTION('center_axis',(-0.173648177666903,0.,-0.984807753012213));
#89532=DIRECTION('ref_axis',(-0.984807753012213,0.,0.173648177666903));
#89533=DIRECTION('center_axis',(0.173648177666902,0.,0.984807753012213));
#89534=DIRECTION('ref_axis',(0.984807753012213,0.,-0.173648177666902));
#89535=DIRECTION('center_axis',(-0.173648177666902,0.,-0.984807753012213));
#89536=DIRECTION('ref_axis',(0.984807753012213,0.,-0.173648177666902));
#89537=DIRECTION('',(-0.173648177666902,0.,-0.984807753012213));
#89538=DIRECTION('center_axis',(0.173648177666902,0.,0.984807753012213));
#89539=DIRECTION('ref_axis',(-0.984807753012213,0.,0.173648177666902));
#89540=DIRECTION('center_axis',(0.173648177666902,0.,0.984807753012213));
#89541=DIRECTION('ref_axis',(-0.984807753012213,0.,0.173648177666902));
#89542=DIRECTION('center_axis',(0.173648177666902,0.,0.984807753012213));
#89543=DIRECTION('ref_axis',(0.984807753012213,0.,-0.173648177666902));
#89544=DIRECTION('center_axis',(0.173648177666902,0.,0.984807753012213));
#89545=DIRECTION('ref_axis',(0.984807753012213,0.,-0.173648177666902));
#89546=DIRECTION('center_axis',(1.2060416625019E-16,-1.,-2.12657684957542E-17));
#89547=DIRECTION('ref_axis',(-0.984807753012213,-1.22464679914735E-16,0.173648177666902));
#89548=DIRECTION('center_axis',(-0.173648177666902,0.,-0.984807753012213));
#89549=DIRECTION('ref_axis',(-0.984807753012213,0.,0.173648177666902));
#89550=DIRECTION('center_axis',(-0.173648177666902,0.,-0.984807753012213));
#89551=DIRECTION('ref_axis',(-0.984807753012213,0.,0.173648177666902));
#89552=DIRECTION('center_axis',(-1.2060416625019E-16,-1.,2.12657684957543E-17));
#89553=DIRECTION('ref_axis',(0.984807753012213,-1.22464679914735E-16,-0.173648177666902));
#89554=DIRECTION('center_axis',(-0.173648177666902,0.,-0.984807753012213));
#89555=DIRECTION('ref_axis',(-0.984807753012213,0.,0.173648177666902));
#89556=DIRECTION('center_axis',(1.2060416625019E-16,1.,-2.12657684957543E-17));
#89557=DIRECTION('ref_axis',(0.984807753012213,-1.22464679914735E-16,-0.173648177666902));
#89558=DIRECTION('center_axis',(0.173648177666902,0.,0.984807753012213));
#89559=DIRECTION('ref_axis',(0.984807753012213,0.,-0.173648177666902));
#89560=DIRECTION('center_axis',(0.173648177666902,0.,0.984807753012213));
#89561=DIRECTION('ref_axis',(0.984807753012213,0.,-0.173648177666902));
#89562=DIRECTION('',(0.173648177666902,0.,0.984807753012213));
#89563=DIRECTION('center_axis',(0.173648177666902,0.,0.984807753012213));
#89564=DIRECTION('ref_axis',(0.984807753012213,0.,-0.173648177666902));
#89565=DIRECTION('center_axis',(0.173648177666902,0.,0.984807753012213));
#89566=DIRECTION('ref_axis',(0.984807753012213,0.,-0.173648177666902));
#89567=DIRECTION('center_axis',(-1.2060416625019E-16,1.,2.12657684957542E-17));
#89568=DIRECTION('ref_axis',(-0.984807753012213,-1.22464679914735E-16,0.173648177666903));
#89569=DIRECTION('center_axis',(-0.173648177666902,0.,-0.984807753012213));
#89570=DIRECTION('ref_axis',(0.984807753012213,0.,-0.173648177666902));
#89571=DIRECTION('center_axis',(-0.173648177666904,0.,-0.984807753012213));
#89572=DIRECTION('ref_axis',(-0.984807753012213,0.,0.173648177666904));
#89573=DIRECTION('center_axis',(-0.173648177666904,0.,-0.984807753012213));
#89574=DIRECTION('ref_axis',(-0.984807753012213,0.,0.173648177666904));
#89575=DIRECTION('',(0.173648177666904,0.,0.984807753012213));
#89576=DIRECTION('center_axis',(-0.173648177666904,0.,-0.984807753012213));
#89577=DIRECTION('ref_axis',(-0.984807753012213,0.,0.173648177666904));
#89578=DIRECTION('center_axis',(0.173648177666884,0.,0.984807753012216));
#89579=DIRECTION('ref_axis',(0.984807753012216,0.,-0.173648177666884));
#89580=DIRECTION('center_axis',(-0.173648177666902,0.,-0.984807753012213));
#89581=DIRECTION('ref_axis',(-0.984807753012213,0.,0.173648177666902));
#89582=DIRECTION('',(-0.173648177666884,0.,-0.984807753012216));
#89583=DIRECTION('center_axis',(0.173648177666884,0.,0.984807753012216));
#89584=DIRECTION('ref_axis',(0.984807753012216,0.,-0.173648177666884));
#89585=DIRECTION('center_axis',(-0.173648177666902,0.,-0.984807753012213));
#89586=DIRECTION('ref_axis',(-0.984807753012213,0.,0.173648177666902));
#89587=DIRECTION('center_axis',(0.173648177666902,0.,0.984807753012213));
#89588=DIRECTION('ref_axis',(0.,-1.,0.));
#89589=DIRECTION('center_axis',(0.173648177666902,0.,0.984807753012213));
#89590=DIRECTION('ref_axis',(0.,-1.,0.));
#89591=DIRECTION('center_axis',(-0.173648177666902,0.,-0.984807753012213));
#89592=DIRECTION('ref_axis',(-0.984807753012213,0.,0.173648177666902));
#89593=DIRECTION('center_axis',(-0.173648177666884,0.,-0.984807753012216));
#89594=DIRECTION('ref_axis',(-0.984807753012216,0.,0.173648177666884));
#89595=DIRECTION('center_axis',(0.173648177666884,0.,0.984807753012216));
#89596=DIRECTION('ref_axis',(0.984807753012216,0.,-0.173648177666884));
#89597=DIRECTION('center_axis',(-0.173648177666902,0.,-0.984807753012213));
#89598=DIRECTION('ref_axis',(-0.984807753012213,0.,0.173648177666902));
#89599=DIRECTION('',(0.171010071662808,-0.984807753012213,-0.0301536896070361));
#89600=DIRECTION('center_axis',(-0.969846310392964,-0.173648177666903,0.171010071662808));
#89601=DIRECTION('ref_axis',(-0.176244384228223,0.984346441568219,-1.7290608322831E-18));
#89602=DIRECTION('',(0.171010071662808,-0.984807753012213,-0.0301536896070361));
#89603=DIRECTION('center_axis',(-0.173648177666902,0.,-0.984807753012213));
#89604=DIRECTION('ref_axis',(-0.984807753012213,0.,0.173648177666902));
#89605=DIRECTION('',(-0.171010071662808,0.984807753012213,0.0301536896070361));
#89606=DIRECTION('center_axis',(0.969846310392964,0.173648177666903,-0.171010071662808));
#89607=DIRECTION('ref_axis',(2.6217127112405E-18,-0.701673843159865,-0.712498293208669));
#89608=DIRECTION('',(-0.171010071662808,0.984807753012213,0.0301536896070361));
#89609=DIRECTION('center_axis',(0.173648177666902,0.,0.984807753012213));
#89610=DIRECTION('ref_axis',(0.,-1.,0.));
#89611=DIRECTION('center_axis',(-0.173648177666902,0.,-0.984807753012213));
#89612=DIRECTION('ref_axis',(-0.984807753012213,0.,0.173648177666902));
#89613=DIRECTION('center_axis',(-0.173648177666902,0.,-0.984807753012213));
#89614=DIRECTION('ref_axis',(-0.984807753012213,0.,0.173648177666902));
#89615=DIRECTION('center_axis',(-0.173648177666902,2.26576127474522E-17,
-0.984807753012213));
#89616=DIRECTION('ref_axis',(0.17101007166281,-0.984807753012213,-0.0301536896070364));
#89617=DIRECTION('center_axis',(0.173648177666902,-7.67302066723185E-16,
0.984807753012213));
#89618=DIRECTION('ref_axis',(0.171010071662807,-0.984807753012213,-0.0301536896070368));
#89619=DIRECTION('center_axis',(0.173648177666902,0.,0.984807753012213));
#89620=DIRECTION('ref_axis',(0.,-1.,0.));
#181110=CARTESIAN_POINT('',(0.,0.,0.));
#181111=CARTESIAN_POINT('Origin',(80.4848979285703,-6.7762635780344E-18,
101.037257330549));
#181112=CARTESIAN_POINT('',(78.7746251576811,2.44276330247173E-16,103.143297948862));
#181113=CARTESIAN_POINT('Origin',(80.7934810513561,-6.7762635780344E-18,
102.787319184645));
#181114=CARTESIAN_POINT('',(79.3342829232298,-6.7762635780344E-18,106.317274859827));
#181115=CARTESIAN_POINT('',(78.4660420348953,-2.57828857403242E-16,101.393236094766));
#181116=CARTESIAN_POINT('',(83.3719947105798,-2.57828857403242E-16,105.605317331393));
#181117=CARTESIAN_POINT('Origin',(81.3531388169048,-6.7762635780344E-18,
105.96129609561));
#181118=CARTESIAN_POINT('Origin',(81.3531388169048,-6.7762635780344E-18,
105.96129609561));
#181119=CARTESIAN_POINT('Origin',(81.3531388169048,-6.7762635780344E-18,
105.96129609561));
#181120=CARTESIAN_POINT('',(81.5670324381031,-6.7762635780344E-18,107.174347100844));
#181121=CARTESIAN_POINT('',(83.3719947105798,-2.57828857403242E-16,105.605317331393));
#181122=CARTESIAN_POINT('Origin',(83.3215010572291,0.,102.341561049839));
#181123=CARTESIAN_POINT('Origin',(76.0518331668413,7.15881389286582E-15,
75.8960977421633));
#181124=CARTESIAN_POINT('',(75.2620568904884,5.41644264137289,76.9170539108621));
#181125=CARTESIAN_POINT('',(75.2383357389536,5.41644264172234,76.7825245640101));
#181126=CARTESIAN_POINT('',(75.1112777726958,5.41644264156718,76.061943035002));
#181127=CARTESIAN_POINT('',(74.0817004664548,-5.09516704230596,76.6496559375717));
#181128=CARTESIAN_POINT('Ctrl Pts',(75.2620568894032,5.4164426411786,76.9170539110535));
#181129=CARTESIAN_POINT('Ctrl Pts',(75.2754748959648,5.4188551225797,76.9143605053861));
#181130=CARTESIAN_POINT('Ctrl Pts',(75.28890236133,5.42121578956793,76.9116672629974));
#181131=CARTESIAN_POINT('Ctrl Pts',(75.3498183865431,5.43168291146175,76.899457787892));
#181132=CARTESIAN_POINT('Ctrl Pts',(75.397407342647,5.43919276600061,76.8899439198397));
#181133=CARTESIAN_POINT('Ctrl Pts',(75.5691587465013,5.46389865606945,76.8556799658338));
#181134=CARTESIAN_POINT('Ctrl Pts',(75.6938224042956,5.47733403583914,76.8309446188927));
#181135=CARTESIAN_POINT('Ctrl Pts',(76.0833251774047,5.50537123701008,76.753856710618));
#181136=CARTESIAN_POINT('Ctrl Pts',(76.3488690788813,5.50451815465259,76.7015654343039));
#181137=CARTESIAN_POINT('Ctrl Pts',(76.7819677492927,5.47054359542805,76.6158738562889));
#181138=CARTESIAN_POINT('Ctrl Pts',(76.9499775446775,5.44922571831477,76.5825354314886));
#181139=CARTESIAN_POINT('Ctrl Pts',(77.1989725367566,5.40542361949064,76.5328721896949));
#181140=CARTESIAN_POINT('Ctrl Pts',(77.2809009315948,5.38900486053439,76.5164900632926));
#181141=CARTESIAN_POINT('Ctrl Pts',(77.4319656140279,5.35499689484238,76.4861991522373));
#181142=CARTESIAN_POINT('Ctrl Pts',(77.5011997889919,5.33793639829778,76.4722832561289));
#181143=CARTESIAN_POINT('Ctrl Pts',(77.6607876106394,5.29517947399735,76.4401268178773));
#181144=CARTESIAN_POINT('Ctrl Pts',(77.7508508200501,5.2684672559417,76.421919232507));
#181145=CARTESIAN_POINT('Ctrl Pts',(77.9445111262649,5.2053902053854,76.3826415096026));
#181146=CARTESIAN_POINT('Ctrl Pts',(78.047793549123,5.16817231010113,76.3616135718207));
#181147=CARTESIAN_POINT('Ctrl Pts',(78.3982901530972,5.02946474761941,76.2900156163008));
#181148=CARTESIAN_POINT('Ctrl Pts',(78.6391363859982,4.91250429236052,76.2403820339988));
#181149=CARTESIAN_POINT('Ctrl Pts',(78.9640140544602,4.72343265372075,76.1733340345982));
#181150=CARTESIAN_POINT('Ctrl Pts',(79.0559021677069,4.6661656823457,76.1543616728065));
#181151=CARTESIAN_POINT('Ctrl Pts',(79.1876829550696,4.57840398389198,76.1271934223636));
#181152=CARTESIAN_POINT('Ctrl Pts',(79.2289357318011,4.55009352929507,76.1186948027529));
#181153=CARTESIAN_POINT('Ctrl Pts',(79.3045197382148,4.49666034899782,76.1031423463777));
#181154=CARTESIAN_POINT('Ctrl Pts',(79.33895565857,4.47170091527016,76.096064838527));
#181155=CARTESIAN_POINT('Ctrl Pts',(79.4306514898834,4.40357217899605,76.0772348049118));
#181156=CARTESIAN_POINT('Ctrl Pts',(79.4873689460504,4.35965364456593,76.0656040707921));
#181157=CARTESIAN_POINT('Ctrl Pts',(79.6190281180506,4.25344678811769,76.0386127554299));
#181158=CARTESIAN_POINT('Ctrl Pts',(79.6932142045313,4.19022250696668,76.0234095759825));
#181159=CARTESIAN_POINT('Ctrl Pts',(80.0374156191236,3.88045569768894,75.9527511024005));
#181160=CARTESIAN_POINT('Ctrl Pts',(80.2842085570211,3.60858291369714,75.901651476153));
#181161=CARTESIAN_POINT('Ctrl Pts',(80.5538836436764,3.24344014059142,75.8438652635243));
#181162=CARTESIAN_POINT('Ctrl Pts',(80.6039551022752,3.17213362785322,75.833039699647));
#181163=CARTESIAN_POINT('Ctrl Pts',(80.6918533153087,3.04036572112086,75.8138438069116));
#181164=CARTESIAN_POINT('Ctrl Pts',(80.7302383807383,2.98031315297712,75.805387912181));
#181165=CARTESIAN_POINT('Ctrl Pts',(80.8149271718713,2.84193599131267,75.7865565325153));
#181166=CARTESIAN_POINT('Ctrl Pts',(80.8604814075452,2.76316206775251,75.776297729902));
#181167=CARTESIAN_POINT('Ctrl Pts',(81.0353628071834,2.4426031910518,75.7363740307411));
#181168=CARTESIAN_POINT('Ctrl Pts',(81.1485813520934,2.19217891526517,75.7092258917502));
#181169=CARTESIAN_POINT('Ctrl Pts',(81.3286618770366,1.69898218475199,75.6635929150326));
#181170=CARTESIAN_POINT('Ctrl Pts',(81.3985430044552,1.45808072721642,75.6446119749557));
#181171=CARTESIAN_POINT('Ctrl Pts',(81.464836328048,1.15442628172622,75.6251491710594));
#181172=CARTESIAN_POINT('Ctrl Pts',(81.4767001255558,1.0955439347704,75.6215788870083));
#181173=CARTESIAN_POINT('Ctrl Pts',(81.494706390344,0.998097598559453,75.6160158592297));
#181174=CARTESIAN_POINT('Ctrl Pts',(81.501396495175,0.959646541580208,75.6139091227582));
#181175=CARTESIAN_POINT('Ctrl Pts',(81.5153461757035,0.87419372173092,75.6094250171015));
#181176=CARTESIAN_POINT('Ctrl Pts',(81.5224104509144,0.827162092638322,
75.6070883012019));
#181177=CARTESIAN_POINT('Ctrl Pts',(81.5444776036597,0.666321761140413,
75.5995310612406));
#181178=CARTESIAN_POINT('Ctrl Pts',(81.5565842571607,0.552118721185883,
75.5949037411769));
#181179=CARTESIAN_POINT('Ctrl Pts',(81.5811858603854,0.223914095366242,
75.5835685654046));
#181180=CARTESIAN_POINT('Ctrl Pts',(81.5849165887661,0.00941249962848681,
75.5785328573369));
#181181=CARTESIAN_POINT('Ctrl Pts',(81.5669627093228,-0.436628439375698,
75.5724285508419));
#181182=CARTESIAN_POINT('Ctrl Pts',(81.5431824625473,-0.667666921105809,
75.5717225500968));
#181183=CARTESIAN_POINT('Ctrl Pts',(81.4903615978844,-0.984792113831477,
75.5738885047287));
#181184=CARTESIAN_POINT('Ctrl Pts',(81.4735382064467,-1.07267417905273,
75.5748299440397));
#181185=CARTESIAN_POINT('Ctrl Pts',(81.4392804126417,-1.23087722059542,
75.5771350847878));
#181186=CARTESIAN_POINT('Ctrl Pts',(81.4225770648942,-1.30133700978203,
75.5783839377358));
#181187=CARTESIAN_POINT('Ctrl Pts',(81.3820113412801,-1.45870533700053,
75.5816717052041));
#181188=CARTESIAN_POINT('Ctrl Pts',(81.357403390545,-1.54539764611939,75.5838285392543));
#181189=CARTESIAN_POINT('Ctrl Pts',(81.3004508501523,-1.72894093691882,
75.5891397869368));
#181190=CARTESIAN_POINT('Ctrl Pts',(81.267523611845,-1.82557326085189,75.5923876027384));
#181191=CARTESIAN_POINT('Ctrl Pts',(81.1571132433896,-2.12255911783891,
75.6038073507318));
#181192=CARTESIAN_POINT('Ctrl Pts',(81.0706849500237,-2.31931492465621,
75.6134387538996));
#181193=CARTESIAN_POINT('Ctrl Pts',(80.8909345968818,-2.67162652378668,
75.6348655220105));
#181194=CARTESIAN_POINT('Ctrl Pts',(80.8009360595584,-2.82858838624564,
75.6460731196286));
#181195=CARTESIAN_POINT('Ctrl Pts',(80.6744272125664,-3.02622880126914,
75.6625920261535));
#181196=CARTESIAN_POINT('Ctrl Pts',(80.6446910284241,-3.07122708385836,
75.6665235973506));
#181197=CARTESIAN_POINT('Ctrl Pts',(80.5908504064156,-3.15017733247058,
75.6737350203911));
#181198=CARTESIAN_POINT('Ctrl Pts',(80.5670090336757,-3.18430657813894,
75.6769596532948));
#181199=CARTESIAN_POINT('Ctrl Pts',(80.505795028728,-3.26986786533731,75.6853142290436));
#181200=CARTESIAN_POINT('Ctrl Pts',(80.467923522806,-3.32092356857916,75.6905502345333));
#181201=CARTESIAN_POINT('Ctrl Pts',(80.3797407701987,-3.43562197010435,
75.7028708998814));
#181202=CARTESIAN_POINT('Ctrl Pts',(80.3288975903319,-3.4988249462727,75.7100646514684));
#181203=CARTESIAN_POINT('Ctrl Pts',(80.1361461507751,-3.72790334146643,
75.737594675469));
#181204=CARTESIAN_POINT('Ctrl Pts',(79.9859162441715,-3.88631031285377,
75.7595368878297));
#181205=CARTESIAN_POINT('Ctrl Pts',(79.6887002358404,-4.16442701220919,
75.8032680716101));
#181206=CARTESIAN_POINT('Ctrl Pts',(79.5441271611145,-4.28629294341588,
75.8246627276548));
#181207=CARTESIAN_POINT('Ctrl Pts',(79.3256304547381,-4.45185119459827,
75.8570015179661));
#181208=CARTESIAN_POINT('Ctrl Pts',(79.2564754918251,-4.50173872972957,
75.8672384238845));
#181209=CARTESIAN_POINT('Ctrl Pts',(79.1267894576786,-4.59073528490751,
75.8864280788308));
#181210=CARTESIAN_POINT('Ctrl Pts',(79.066593275645,-4.63030858391227,75.8953324794358));
#181211=CARTESIAN_POINT('Ctrl Pts',(78.9263188117953,-4.71858278959934,
75.916072038791));
#181212=CARTESIAN_POINT('Ctrl Pts',(78.8457387544382,-4.76642607583487,
75.9279781728946));
#181213=CARTESIAN_POINT('Ctrl Pts',(78.5423740529721,-4.93607949645029,
75.9727756950506));
#181214=CARTESIAN_POINT('Ctrl Pts',(78.3124722047592,-5.04422621065495,
76.0066565681112));
#181215=CARTESIAN_POINT('Ctrl Pts',(77.829034184455,-5.23142919103745,76.0781259275798));
#181216=CARTESIAN_POINT('Ctrl Pts',(77.57553792995,-5.30874219937458,76.1157201246387));
#181217=CARTESIAN_POINT('Ctrl Pts',(77.2613744437602,-5.37984977586853,
76.1630056636212));
#181218=CARTESIAN_POINT('Ctrl Pts',(77.2049732316613,-5.39166898964449,
76.171522191863));
#181219=CARTESIAN_POINT('Ctrl Pts',(77.1106473714662,-5.40986282727492,
76.185820895061));
#181220=CARTESIAN_POINT('Ctrl Pts',(77.0728198473076,-5.41674027081251,
76.1915702330033));
#181221=CARTESIAN_POINT('Ctrl Pts',(76.9874458561194,-5.43132033513407,
76.2045818145711));
#181222=CARTESIAN_POINT('Ctrl Pts',(76.9398661403242,-5.43879081781303,
76.2118571995347));
#181223=CARTESIAN_POINT('Ctrl Pts',(76.7707178504184,-5.46302850165962,
76.2377912634859));
#181224=CARTESIAN_POINT('Ctrl Pts',(76.6487101659722,-5.47627255080551,
76.2566244422886));
#181225=CARTESIAN_POINT('Ctrl Pts',(76.2772451744542,-5.50377573338375,
76.3141500007427));
#181226=CARTESIAN_POINT('Ctrl Pts',(76.0271968622321,-5.50482793264817,
76.3531135380574));
#181227=CARTESIAN_POINT('Ctrl Pts',(75.5904385492959,-5.47618087078442,
76.4208474296114));
#181228=CARTESIAN_POINT('Ctrl Pts',(75.4036881002443,-5.45405748105691,
76.449707646761));
#181229=CARTESIAN_POINT('Ctrl Pts',(75.134044336607,-5.40769034260733,76.4910798024161));
#181230=CARTESIAN_POINT('Ctrl Pts',(75.0500205098195,-5.39117040414606,
76.5039299457892));
#181231=CARTESIAN_POINT('Ctrl Pts',(74.8963813196968,-5.35714187775381,
76.5273409156258));
#181232=CARTESIAN_POINT('Ctrl Pts',(74.8266578676524,-5.34023319653329,
76.5379322689636));
#181233=CARTESIAN_POINT('Ctrl Pts',(74.6899154236981,-5.3041696216234,76.5586372141246));
#181234=CARTESIAN_POINT('Ctrl Pts',(74.6228894075215,-5.28509750715447,
76.5687538291483));
#181235=CARTESIAN_POINT('Ctrl Pts',(74.395584105041,-5.21563647174156,76.6029539396097));
#181236=CARTESIAN_POINT('Ctrl Pts',(74.2372332825469,-5.15905477625702,
76.6265903536784));
#181237=CARTESIAN_POINT('Ctrl Pts',(74.0817004664548,-5.09516704230593,
76.6496559375717));
#181238=CARTESIAN_POINT('',(79.7540569593757,-4.07954801327269,75.649466443673));
#181239=CARTESIAN_POINT('Origin',(76.1212924379081,7.15881389286582E-15,
76.2900208433682));
#181240=CARTESIAN_POINT('Ctrl Pts',(79.7540569593757,-4.07954801327269,
75.649466443673));
#181241=CARTESIAN_POINT('Ctrl Pts',(79.9550556064584,-3.89610083871904,
75.6210523034932));
#181242=CARTESIAN_POINT('Ctrl Pts',(80.1423230216256,-3.69778482906888,
75.5952486961923));
#181243=CARTESIAN_POINT('Ctrl Pts',(80.3562343526423,-3.43456767337074,
75.5661552350339));
#181244=CARTESIAN_POINT('Ctrl Pts',(80.3972895896231,-3.382133321999,75.5605900939294));
#181245=CARTESIAN_POINT('Ctrl Pts',(80.4707099816455,-3.2847719269421,75.5506576046304));
#181246=CARTESIAN_POINT('Ctrl Pts',(80.5033667439126,-3.24007982786696,
75.5462473578158));
#181247=CARTESIAN_POINT('Ctrl Pts',(80.5596008253803,-3.16063129437193,
75.5386577661436));
#181248=CARTESIAN_POINT('Ctrl Pts',(80.5834624070778,-3.12608747664255,
75.5354381457118));
#181249=CARTESIAN_POINT('Ctrl Pts',(80.6363530629559,-3.04761418133183,
75.5283058804656));
#181250=CARTESIAN_POINT('Ctrl Pts',(80.6651527602619,-3.00353353717,75.524426001573));
#181251=CARTESIAN_POINT('Ctrl Pts',(80.8478409371821,-2.71496953037959,
75.4998728557273));
#181252=CARTESIAN_POINT('Ctrl Pts',(80.9830572573553,-2.45897192043341,
75.482000099418));
#181253=CARTESIAN_POINT('Ctrl Pts',(81.1823475989033,-1.99788564595248,
75.4574826058732));
#181254=CARTESIAN_POINT('Ctrl Pts',(81.2556070490208,-1.79756030707335,
75.4491368303146));
#181255=CARTESIAN_POINT('Ctrl Pts',(81.3420230087736,-1.51152230905519,
75.4406024945352));
#181256=CARTESIAN_POINT('Ctrl Pts',(81.3648982333203,-1.42900607922151,
75.4385212107493));
#181257=CARTESIAN_POINT('Ctrl Pts',(81.4036544248634,-1.27561407896006,
75.4353608550889));
#181258=CARTESIAN_POINT('Ctrl Pts',(81.4200661527256,-1.20489424898321,
75.434177700621));
#181259=CARTESIAN_POINT('Ctrl Pts',(81.4543841896188,-1.04276060042251,
75.4320910447137));
#181260=CARTESIAN_POINT('Ctrl Pts',(81.4713946674952,-0.951177810721096,
75.4313617794898));
#181261=CARTESIAN_POINT('Ctrl Pts',(81.536412068738,-0.544957176818441,
75.430100047732));
#181262=CARTESIAN_POINT('Ctrl Pts',(81.5598456418334,-0.226990638240277,
75.4343482823491));
#181263=CARTESIAN_POINT('Ctrl Pts',(81.5535579234438,0.305419715144901,
75.449484331721));
#181264=CARTESIAN_POINT('Ctrl Pts',(81.5386878444932,0.519344982180364,
75.4577279527938));
#181265=CARTESIAN_POINT('Ctrl Pts',(81.5046293544219,0.785579410276051,
75.4703960790198));
#181266=CARTESIAN_POINT('Ctrl Pts',(81.4969606121235,0.839262145573826,
75.4730741056276));
#181267=CARTESIAN_POINT('Ctrl Pts',(81.482495066884,0.930896376042242,75.4778492770305));
#181268=CARTESIAN_POINT('Ctrl Pts',(81.4760872172513,0.968907308844052,
75.4798900109912));
#181269=CARTESIAN_POINT('Ctrl Pts',(81.460350056275,1.05665918084017,75.4847398795328));
#181270=CARTESIAN_POINT('Ctrl Pts',(81.4507352996072,1.10634194800698,75.4875901851627));
#181271=CARTESIAN_POINT('Ctrl Pts',(81.4135605586294,1.28526291080719,75.4982497703578));
#181272=CARTESIAN_POINT('Ctrl Pts',(81.3820665205496,1.41360171289019,75.5066444834221));
#181273=CARTESIAN_POINT('Ctrl Pts',(81.2853833688129,1.75449848831423,75.5311718921765));
#181274=CARTESIAN_POINT('Ctrl Pts',(81.2119666585506,1.96436331166959,75.5486561367009));
#181275=CARTESIAN_POINT('Ctrl Pts',(81.0469581347712,2.35840784715467,75.5867078861355));
#181276=CARTESIAN_POINT('Ctrl Pts',(80.9572801169381,2.54301636247878,75.6069141242577));
#181277=CARTESIAN_POINT('Ctrl Pts',(80.8158730901985,2.79710961068029,75.6383745935883));
#181278=CARTESIAN_POINT('Ctrl Pts',(80.7723632254629,2.87116481313088,75.6480087669995));
#181279=CARTESIAN_POINT('Ctrl Pts',(80.6892237466168,3.00538436733356,75.6663453150252));
#181280=CARTESIAN_POINT('Ctrl Pts',(80.6501029267193,3.06585474170003,75.6749466540032));
#181281=CARTESIAN_POINT('Ctrl Pts',(80.5586199607333,3.20134874172161,75.69500380147));
#181282=CARTESIAN_POINT('Ctrl Pts',(80.5055576271492,3.27585249528855,75.70659829089));
#181283=CARTESIAN_POINT('Ctrl Pts',(80.3153733318279,3.52922093305338,75.7480178038986));
#181284=CARTESIAN_POINT('Ctrl Pts',(80.1692329927724,3.70073220098829,75.7796229922203));
#181285=CARTESIAN_POINT('Ctrl Pts',(79.8912362588521,3.9887375940513,75.8391393499741));
#181286=CARTESIAN_POINT('Ctrl Pts',(79.7634556847928,4.10887402418649,75.8662988014842));
#181287=CARTESIAN_POINT('Ctrl Pts',(79.5745540055725,4.26989973790512,75.9060090474467));
#181288=CARTESIAN_POINT('Ctrl Pts',(79.5180016410818,4.31615484337398,75.9178448610913));
#181289=CARTESIAN_POINT('Ctrl Pts',(79.4142133639953,4.397574951187,75.9394533755029));
#181290=CARTESIAN_POINT('Ctrl Pts',(79.367301737562,4.43314718220199,75.9491801320532));
#181291=CARTESIAN_POINT('Ctrl Pts',(79.2864498579615,4.49238704884988,75.9658657738151));
#181292=CARTESIAN_POINT('Ctrl Pts',(79.2527991771433,4.51644961727751,75.9727872746673));
#181293=CARTESIAN_POINT('Ctrl Pts',(79.1714399308616,4.5732161079938,75.9894671128365));
#181294=CARTESIAN_POINT('Ctrl Pts',(79.1234793193192,4.60553833401426,75.9992567928688));
#181295=CARTESIAN_POINT('Ctrl Pts',(78.8770000517463,4.76591235420394,76.0493886449357));
#181296=CARTESIAN_POINT('Ctrl Pts',(78.670842711567,4.88141817520882,76.0907471250219));
#181297=CARTESIAN_POINT('Ctrl Pts',(78.2367696882436,5.08821168409858,76.1775656977172));
#181298=CARTESIAN_POINT('Ctrl Pts',(78.0088279413494,5.17814608798127,76.2230256174725));
#181299=CARTESIAN_POINT('Ctrl Pts',(77.6911731584347,5.27883551707747,76.2866039634875));
#181300=CARTESIAN_POINT('Ctrl Pts',(77.6059881237611,5.30351054739958,76.3036731028311));
#181301=CARTESIAN_POINT('Ctrl Pts',(77.4514940464848,5.34410114405924,76.3346776955947));
#181302=CARTESIAN_POINT('Ctrl Pts',(77.3823972277283,5.36077965847882,76.3485611405648));
#181303=CARTESIAN_POINT('Ctrl Pts',(77.2274214007911,5.39490906576752,76.3797414543912));
#181304=CARTESIAN_POINT('Ctrl Pts',(77.1414099253904,5.41162784306611,76.3970747006309));
#181305=CARTESIAN_POINT('Ctrl Pts',(76.8405040792983,5.46241168766167,76.4578121043415));
#181306=CARTESIAN_POINT('Ctrl Pts',(76.6240506280537,5.48535153572426,76.5016856039424));
#181307=CARTESIAN_POINT('Ctrl Pts',(76.1891201938785,5.50447128643675,76.5900118497044));
#181308=CARTESIAN_POINT('Ctrl Pts',(75.9710362730251,5.50056825728675,76.6343839354773));
#181309=CARTESIAN_POINT('Ctrl Pts',(75.639462516768,5.47408226077514,76.7016256038782));
#181310=CARTESIAN_POINT('Ctrl Pts',(75.5254715132157,5.4612361921884,76.7247000444197));
#181311=CARTESIAN_POINT('Ctrl Pts',(75.3654979479876,5.43792360047614,76.7569585898209));
#181312=CARTESIAN_POINT('Ctrl Pts',(75.3191290837197,5.43053577677619,76.7662939744724));
#181313=CARTESIAN_POINT('Ctrl Pts',(75.2613436702706,5.42054010557266,76.7779049741604));
#181314=CARTESIAN_POINT('Ctrl Pts',(75.2498364807966,5.4185104098025,76.780216012227));
#181315=CARTESIAN_POINT('Ctrl Pts',(75.2383357398202,5.41644264187749,76.7825245638573));
#181316=CARTESIAN_POINT('Origin',(76.0518331668413,7.15881389286582E-15,
75.8960977421633));
#181317=CARTESIAN_POINT('',(75.4009754336961,5.41644264156684,77.7049001130299));
#181318=CARTESIAN_POINT('',(75.3772542814629,5.41644264179018,77.5703707663353));
#181319=CARTESIAN_POINT('',(75.1112777726958,5.41644264156718,76.061943035002));
#181320=CARTESIAN_POINT('Ctrl Pts',(75.4009754336941,5.41644264156649,77.7049001130302));
#181321=CARTESIAN_POINT('Ctrl Pts',(75.4020729769854,5.41663997361865,77.704679802412));
#181322=CARTESIAN_POINT('Ctrl Pts',(75.4031705837651,5.41683695903492,77.7044594928459));
#181323=CARTESIAN_POINT('Ctrl Pts',(75.4452787908983,5.42438030488838,77.696008139894));
#181324=CARTESIAN_POINT('Ctrl Pts',(75.4863750017577,5.43124262170462,77.6877790728472));
#181325=CARTESIAN_POINT('Ctrl Pts',(75.6058154563448,5.44974047445724,77.6639096767692));
#181326=CARTESIAN_POINT('Ctrl Pts',(75.684346011331,5.46010407979348,77.6482745253597));
#181327=CARTESIAN_POINT('Ctrl Pts',(76.1815405376581,5.514400969188,77.5495361110557));
#181328=CARTESIAN_POINT('Ctrl Pts',(76.6039855001008,5.51004359234611,77.466636795253));
#181329=CARTESIAN_POINT('Ctrl Pts',(77.1376747354864,5.44058675271276,77.3606483411415));
#181330=CARTESIAN_POINT('Ctrl Pts',(77.2533426158265,5.4216121665109,77.337609825817));
#181331=CARTESIAN_POINT('Ctrl Pts',(77.4411559288904,5.38436680411922,77.3000613183583));
#181332=CARTESIAN_POINT('Ctrl Pts',(77.5137078564261,5.36838679584465,77.2855219480806));
#181333=CARTESIAN_POINT('Ctrl Pts',(77.6591786277079,5.33312432675046,77.256295596882));
#181334=CARTESIAN_POINT('Ctrl Pts',(77.7320707207943,5.31380021265953,77.2416128781552));
#181335=CARTESIAN_POINT('Ctrl Pts',(77.9256686146808,5.25803217267343,77.2025134307304));
#181336=CARTESIAN_POINT('Ctrl Pts',(78.0455467754778,5.21882418249065,77.1781935283756));
#181337=CARTESIAN_POINT('Ctrl Pts',(78.3296723279193,5.11456155376492,77.1203157462599));
#181338=CARTESIAN_POINT('Ctrl Pts',(78.4923367479489,5.04550175049125,77.0869823530995));
#181339=CARTESIAN_POINT('Ctrl Pts',(78.8518658917288,4.87130021871031,77.0130368007182));
#181340=CARTESIAN_POINT('Ctrl Pts',(79.0462544723592,4.7616095652405,76.9728592553762));
#181341=CARTESIAN_POINT('Ctrl Pts',(79.2826381127944,4.60806484841252,76.9241008976943));
#181342=CARTESIAN_POINT('Ctrl Pts',(79.3312901338968,4.57531974836113,76.9140717788956));
#181343=CARTESIAN_POINT('Ctrl Pts',(79.4133424573088,4.51812688394018,76.8971790129097));
#181344=CARTESIAN_POINT('Ctrl Pts',(79.4470046036712,4.49408357014091,76.8902556801653));
#181345=CARTESIAN_POINT('Ctrl Pts',(79.5272278095524,4.43537974882161,76.8737726094502));
#181346=CARTESIAN_POINT('Ctrl Pts',(79.5735201666139,4.40034596551875,76.8642735071764));
#181347=CARTESIAN_POINT('Ctrl Pts',(79.7723850516266,4.24474318335922,76.8234894983546));
#181348=CARTESIAN_POINT('Ctrl Pts',(79.9191117054783,4.11661816826673,76.7934530302152));
#181349=CARTESIAN_POINT('Ctrl Pts',(80.2638622600493,3.78116886457503,76.7224269910616));
#181350=CARTESIAN_POINT('Ctrl Pts',(80.4531485901211,3.56539863205374,76.6829956575978));
#181351=CARTESIAN_POINT('Ctrl Pts',(80.6787780408469,3.26307513276364,76.6347341520628));
#181352=CARTESIAN_POINT('Ctrl Pts',(80.7309999518845,3.18935447349107,76.6234621678859));
#181353=CARTESIAN_POINT('Ctrl Pts',(80.8214803160336,3.0546625416661,76.6037298444661));
#181354=CARTESIAN_POINT('Ctrl Pts',(80.8604024199354,2.9941780035497,76.595167702943));
#181355=CARTESIAN_POINT('Ctrl Pts',(80.9443058915359,2.85796510389816,76.5765371265833));
#181356=CARTESIAN_POINT('Ctrl Pts',(80.988681530533,2.7818746694691,76.566563067203));
#181357=CARTESIAN_POINT('Ctrl Pts',(81.1463780764141,2.49585703268448,76.5306529092568));
#181358=CARTESIAN_POINT('Ctrl Pts',(81.2479050651942,2.2795058314519,76.506559702183));
#181359=CARTESIAN_POINT('Ctrl Pts',(81.442853000442,1.78258182729151,76.4581168680367));
#181360=CARTESIAN_POINT('Ctrl Pts',(81.5285108441798,1.49962495282199,76.4350964575102));
#181361=CARTESIAN_POINT('Ctrl Pts',(81.6041246215021,1.15261992842301,76.4128846558187));
#181362=CARTESIAN_POINT('Ctrl Pts',(81.6158988443021,1.09409238604093,76.4093396837614));
#181363=CARTESIAN_POINT('Ctrl Pts',(81.6338115843297,0.997044222537231,
76.4038036237688));
#181364=CARTESIAN_POINT('Ctrl Pts',(81.6404871299318,0.958634294155849,
76.4017007422951));
#181365=CARTESIAN_POINT('Ctrl Pts',(81.6544464092353,0.873028147085903,
76.3972118927654));
#181366=CARTESIAN_POINT('Ctrl Pts',(81.6615290211364,0.825801121556553,
76.3948677969999));
#181367=CARTESIAN_POINT('Ctrl Pts',(81.683792191991,0.663193268090111,76.3872371519462));
#181368=CARTESIAN_POINT('Ctrl Pts',(81.6959842799855,0.547406690715393,
76.3825624941172));
#181369=CARTESIAN_POINT('Ctrl Pts',(81.7207781897654,0.211548296276864,
76.3710364535082));
#181370=CARTESIAN_POINT('Ctrl Pts',(81.7240070003098,-0.00904462314788024,
76.3659708117056));
#181371=CARTESIAN_POINT('Ctrl Pts',(81.7042080129052,-0.452474710442173,
76.3602340745503));
#181372=CARTESIAN_POINT('Ctrl Pts',(81.6808467751521,-0.674884822386066,
76.3596261769768));
#181373=CARTESIAN_POINT('Ctrl Pts',(81.6294851487584,-0.983685275673139,
76.3617239203034));
#181374=CARTESIAN_POINT('Ctrl Pts',(81.612650234701,-1.07171750319945,76.3626643100358));
#181375=CARTESIAN_POINT('Ctrl Pts',(81.5783843811993,-1.23007142514674,
76.3649678642025));
#181376=CARTESIAN_POINT('Ctrl Pts',(81.5616915987074,-1.30053330021413,
76.3662150605287));
#181377=CARTESIAN_POINT('Ctrl Pts',(81.5211878885947,-1.45775780560969,
76.3694960067721));
#181378=CARTESIAN_POINT('Ctrl Pts',(81.4966385721934,-1.54430627648585,
76.371646540938));
#181379=CARTESIAN_POINT('Ctrl Pts',(81.3954187544674,-1.87077914819239,
76.3810810293745));
#181380=CARTESIAN_POINT('Ctrl Pts',(81.3045982606598,-2.10592696902885,
76.3906096568055));
#181381=CARTESIAN_POINT('Ctrl Pts',(81.0980492338646,-2.54874766688467,
76.4143293583233));
#181382=CARTESIAN_POINT('Ctrl Pts',(80.984299133772,-2.75676566615468,76.4281952746031));
#181383=CARTESIAN_POINT('Ctrl Pts',(80.8263555253881,-3.00632693109112,
76.4487254522299));
#181384=CARTESIAN_POINT('Ctrl Pts',(80.7941999988036,-3.05539644322752,
76.4529623578508));
#181385=CARTESIAN_POINT('Ctrl Pts',(80.7378047895742,-3.13855245758497,
76.4604990868535));
#181386=CARTESIAN_POINT('Ctrl Pts',(80.713943322543,-3.1728950819609,76.4637193241671));
#181387=CARTESIAN_POINT('Ctrl Pts',(80.6553056567348,-3.25528640450156,
76.4717067610597));
#181388=CARTESIAN_POINT('Ctrl Pts',(80.6201469420956,-3.30304696015817,
76.4765552921622));
#181389=CARTESIAN_POINT('Ctrl Pts',(80.5397494552509,-3.40866383795519,
76.4877556768322));
#181390=CARTESIAN_POINT('Ctrl Pts',(80.4941165436365,-3.46619700066956,
76.4941888745555));
#181391=CARTESIAN_POINT('Ctrl Pts',(80.3357899666468,-3.65783274908615,
76.5167148035222));
#181392=CARTESIAN_POINT('Ctrl Pts',(80.2179230208658,-3.78739929961215,
76.5338187546947));
#181393=CARTESIAN_POINT('Ctrl Pts',(79.9325771620297,-4.07241960119109,
76.5755977565229));
#181394=CARTESIAN_POINT('Ctrl Pts',(79.7612179705992,-4.22342178265414,
76.6009428583409));
#181395=CARTESIAN_POINT('Ctrl Pts',(79.508729005858,-4.41923275774376,76.6383078424876));
#181396=CARTESIAN_POINT('Ctrl Pts',(79.4350477229229,-4.47345890814326,
76.6492155511054));
#181397=CARTESIAN_POINT('Ctrl Pts',(79.3010125527878,-4.56698842672564,
76.6690509309088));
#181398=CARTESIAN_POINT('Ctrl Pts',(79.24117105774,-4.60700315214091,76.6779043298694));
#181399=CARTESIAN_POINT('Ctrl Pts',(79.108301688471,-4.69208057689179,76.6975526569854));
#181400=CARTESIAN_POINT('Ctrl Pts',(79.0349697230675,-4.7366222454886,76.7083906944632));
#181401=CARTESIAN_POINT('Ctrl Pts',(78.7829382837485,-4.88164320501621,
76.7456179533184));
#181402=CARTESIAN_POINT('Ctrl Pts',(78.5996839502126,-4.97368642080729,
76.7726433327134));
#181403=CARTESIAN_POINT('Ctrl Pts',(78.2090201216121,-5.14290632603296,
76.8303142993207));
#181404=CARTESIAN_POINT('Ctrl Pts',(78.0012037239324,-5.21818701418991,
76.8610239264968));
#181405=CARTESIAN_POINT('Ctrl Pts',(77.6642970292578,-5.31737531769137,
76.9112002748036));
#181406=CARTESIAN_POINT('Ctrl Pts',(77.5378523013817,-5.34967297348176,
76.930118788903));
#181407=CARTESIAN_POINT('Ctrl Pts',(77.3615192121098,-5.38796516969839,
76.9567074737141));
#181408=CARTESIAN_POINT('Ctrl Pts',(77.3124930965134,-5.39789957191332,
76.9641218116638));
#181409=CARTESIAN_POINT('Ctrl Pts',(77.2258172860334,-5.41421121345534,
76.9772754314374));
#181410=CARTESIAN_POINT('Ctrl Pts',(77.1882232627926,-5.42087336868818,
76.9829960938603));
#181411=CARTESIAN_POINT('Ctrl Pts',(77.0974694270477,-5.43596330120389,
76.996842312823));
#181412=CARTESIAN_POINT('Ctrl Pts',(77.0442524423473,-5.44399427940258,
77.0049905360038));
#181413=CARTESIAN_POINT('Ctrl Pts',(76.7730296211376,-5.48077448131402,
77.0466356050011));
#181414=CARTESIAN_POINT('Ctrl Pts',(76.5536178044252,-5.49693060199017,
77.0807024432229));
#181415=CARTESIAN_POINT('Ctrl Pts',(76.0295409312807,-5.50330296947548,
77.1621358488257));
#181416=CARTESIAN_POINT('Ctrl Pts',(75.7254729986752,-5.48114096815827,
77.2094103944046));
#181417=CARTESIAN_POINT('Ctrl Pts',(75.3331039071907,-5.41878711386261,
77.2697131851974));
#181418=CARTESIAN_POINT('Ctrl Pts',(75.24183316856,-5.40185302300611,77.2836934343694));
#181419=CARTESIAN_POINT('Ctrl Pts',(75.0807363885537,-5.36763604698873,
77.3082732092191));
#181420=CARTESIAN_POINT('Ctrl Pts',(75.0107402169087,-5.35129974146552,
77.3189205734925));
#181421=CARTESIAN_POINT('Ctrl Pts',(74.8594488421186,-5.31278626645264,
77.3418602960457));
#181422=CARTESIAN_POINT('Ctrl Pts',(74.7782993351078,-5.29009305175616,
77.3541177625059));
#181423=CARTESIAN_POINT('Ctrl Pts',(74.5034103532694,-5.20623880419246,
77.3954805960167));
#181424=CARTESIAN_POINT('Ctrl Pts',(74.3125133201331,-5.13603057017492,
77.4239262159174));
#181425=CARTESIAN_POINT('Ctrl Pts',(73.9142066477073,-4.96351707623434,
77.4828457673159));
#181426=CARTESIAN_POINT('Ctrl Pts',(73.7084290046165,-4.85833694299808,
77.513017391783));
#181427=CARTESIAN_POINT('Ctrl Pts',(73.4275874254457,-4.69139566643611,
77.5541776277481));
#181428=CARTESIAN_POINT('Ctrl Pts',(73.3465964460926,-4.64030884468542,
77.5660471991354));
#181429=CARTESIAN_POINT('Ctrl Pts',(73.2283766489362,-4.56129508870328,
77.5834094423849));
#181430=CARTESIAN_POINT('Ctrl Pts',(73.1901007749669,-4.53499711030064,
77.5890367429091));
#181431=CARTESIAN_POINT('Ctrl Pts',(73.1153793664998,-4.48223603124923,
77.6000402064927));
#181432=CARTESIAN_POINT('Ctrl Pts',(73.0789166209474,-4.45580443452335,
77.6054185719554));
#181433=CARTESIAN_POINT('Ctrl Pts',(72.9731907493409,-4.3771434416892,77.6210298216499));
#181434=CARTESIAN_POINT('Ctrl Pts',(72.9048320949972,-4.32369868629183,
77.6311442986488));
#181435=CARTESIAN_POINT('Ctrl Pts',(72.7367403329871,-4.18569092517141,
77.6560110940905));
#181436=CARTESIAN_POINT('Ctrl Pts',(72.6386949300854,-4.09911462700645,
77.6705108504923));
#181437=CARTESIAN_POINT('Ctrl Pts',(72.3221781118181,-3.79876725713764,
77.7170723819862));
#181438=CARTESIAN_POINT('Ctrl Pts',(72.1183040429124,-3.57007414181092,
77.7466130640995));
#181439=CARTESIAN_POINT('Ctrl Pts',(71.8805936079935,-3.25411209035273,
77.7796698119892));
#181440=CARTESIAN_POINT('Ctrl Pts',(71.8286825384416,-3.18152245778924,
77.7867907924351));
#181441=CARTESIAN_POINT('Ctrl Pts',(71.7379596963361,-3.04795473113288,
77.799040617419));
#181442=CARTESIAN_POINT('Ctrl Pts',(71.6985485669373,-2.98741982906312,
77.8042890487759));
#181443=CARTESIAN_POINT('Ctrl Pts',(71.612770761583,-2.84986627949213,77.8155394100314));
#181444=CARTESIAN_POINT('Ctrl Pts',(71.5670652304035,-2.77244937745199,
77.8214110656497));
#181445=CARTESIAN_POINT('Ctrl Pts',(71.4742167268635,-2.60609163312333,
77.8330679582445));
#181446=CARTESIAN_POINT('Ctrl Pts',(71.4275666339812,-2.5169066993107,77.8387576010062));
#181447=CARTESIAN_POINT('Ctrl Pts',(71.2954432723988,-2.2467199983734,77.8543636886155));
#181448=CARTESIAN_POINT('Ctrl Pts',(71.2172493456322,-2.06226476071193,
77.8628851650492));
#181449=CARTESIAN_POINT('Ctrl Pts',(71.0709593663331,-1.6578019620809,77.8773406054602));
#181450=CARTESIAN_POINT('Ctrl Pts',(71.0062029630466,-1.43695961715027,
77.8826913878878));
#181451=CARTESIAN_POINT('Ctrl Pts',(70.9419958661517,-1.15410968631953,
77.8867725233147));
#181452=CARTESIAN_POINT('Ctrl Pts',(70.9296427566043,-1.09528970198231,
77.8874740063728));
#181453=CARTESIAN_POINT('Ctrl Pts',(70.9108368169774,-0.997913445835886,
77.8884038070268));
#181454=CARTESIAN_POINT('Ctrl Pts',(70.9038322756842,-0.959469711642977,
77.8887120344974));
#181455=CARTESIAN_POINT('Ctrl Pts',(70.8891883990514,-0.873990427797152,
77.8892692188217));
#181456=CARTESIAN_POINT('Ctrl Pts',(70.88174751564,-0.82692484798217,77.8894894333077));
#181457=CARTESIAN_POINT('Ctrl Pts',(70.8583903258539,-0.665779445539081,
77.8899350268585));
#181458=CARTESIAN_POINT('Ctrl Pts',(70.8454144177356,-0.551303327335231,
77.8897248713029));
#181459=CARTESIAN_POINT('Ctrl Pts',(70.8183772460396,-0.221792504260873,
77.8874682190748));
#181460=CARTESIAN_POINT('Ctrl Pts',(70.8132260150459,-0.00625418694376014,
77.883978481678));
#181461=CARTESIAN_POINT('Ctrl Pts',(70.8283287089504,0.439340093590735,
77.8720527215784));
#181462=CARTESIAN_POINT('Ctrl Pts',(70.8503748299958,0.668906897706618,
77.8632955563532));
#181463=CARTESIAN_POINT('Ctrl Pts',(70.900513282669,0.984611395727771,77.8473392703025));
#181464=CARTESIAN_POINT('Ctrl Pts',(70.9166457957842,1.07251793677072,77.8424691922593));
#181465=CARTESIAN_POINT('Ctrl Pts',(70.9496271307735,1.23074554550303,77.8329177709531));
#181466=CARTESIAN_POINT('Ctrl Pts',(70.9657485550732,1.30120564917606,77.8283787653097));
#181467=CARTESIAN_POINT('Ctrl Pts',(71.0049824167555,1.45855038017018,77.8175963874491));
#181468=CARTESIAN_POINT('Ctrl Pts',(71.0288346261726,1.54521911779411,77.8112090496226));
#181469=CARTESIAN_POINT('Ctrl Pts',(71.0701833899872,1.68239098540337,77.8003825271014));
#181470=CARTESIAN_POINT('Ctrl Pts',(71.0863337615349,1.73330312264484,77.7962040836166));
#181471=CARTESIAN_POINT('Ctrl Pts',(71.1273534154071,1.85642707029573,77.785710349855));
#181472=CARTESIAN_POINT('Ctrl Pts',(71.1529792845135,1.92836261467522,77.7792503968465));
#181473=CARTESIAN_POINT('Ctrl Pts',(71.2803750611764,2.26390069384434,77.7475803192595));
#181474=CARTESIAN_POINT('Ctrl Pts',(71.4006031665256,2.51970316168431,77.7188925668034));
#181475=CARTESIAN_POINT('Ctrl Pts',(71.5856552511088,2.84570286948372,77.6766585468788));
#181476=CARTESIAN_POINT('Ctrl Pts',(71.6335825210212,2.92534704552493,77.6658586588896));
#181477=CARTESIAN_POINT('Ctrl Pts',(71.710719898781,3.04643591043896,77.6487169441098));
#181478=CARTESIAN_POINT('Ctrl Pts',(71.7385303697219,3.08878084829776,77.6425812864957));
#181479=CARTESIAN_POINT('Ctrl Pts',(71.7908543550672,3.16608269784157,77.6311250739553));
#181480=CARTESIAN_POINT('Ctrl Pts',(71.8151978882991,3.20115246897619,77.6258289927339));
#181481=CARTESIAN_POINT('Ctrl Pts',(71.8813405265814,3.2940896995417,77.6115223418272));
#181482=CARTESIAN_POINT('Ctrl Pts',(71.9238614684829,3.35141741247608,77.6024099501953));
#181483=CARTESIAN_POINT('Ctrl Pts',(72.0264026356097,3.48413774177117,77.5805983463726));
#181484=CARTESIAN_POINT('Ctrl Pts',(72.0873116371339,3.55879082933397,77.5677657761391));
#181485=CARTESIAN_POINT('Ctrl Pts',(72.38187649175,3.90088479971365,77.5061255652904));
#181486=CARTESIAN_POINT('Ctrl Pts',(72.6390036122654,4.14623817745918,77.4534368313759));
#181487=CARTESIAN_POINT('Ctrl Pts',(72.9891238576085,4.4202247383,77.3816818103994));
#181488=CARTESIAN_POINT('Ctrl Pts',(73.0619162488184,4.47428803197506,77.3667672672356));
#181489=CARTESIAN_POINT('Ctrl Pts',(73.1944674744102,4.5676441899567,77.3396015043864));
#181490=CARTESIAN_POINT('Ctrl Pts',(73.253726106972,4.60763905340021,77.3274543564964));
#181491=CARTESIAN_POINT('Ctrl Pts',(73.3854622364641,4.6927802690722,77.3004409126648));
#181492=CARTESIAN_POINT('Ctrl Pts',(73.4582448808783,4.73739770708001,77.2855101356409));
#181493=CARTESIAN_POINT('Ctrl Pts',(73.7099649488329,4.88356583266327,77.2338498438234));
#181494=CARTESIAN_POINT('Ctrl Pts',(73.8935143340935,4.97645774825786,77.1961357341674));
#181495=CARTESIAN_POINT('Ctrl Pts',(74.3858621449977,5.19090980433098,77.095051778343));
#181496=CARTESIAN_POINT('Ctrl Pts',(74.7012287712784,5.29452021051441,77.0303520702087));
#181497=CARTESIAN_POINT('Ctrl Pts',(75.0791751485197,5.38053464508495,76.953875080421));
#181498=CARTESIAN_POINT('Ctrl Pts',(75.1344859300275,5.39219440762119,76.94271022217));
#181499=CARTESIAN_POINT('Ctrl Pts',(75.2139692185283,5.40762470150229,76.9267132106787));
#181500=CARTESIAN_POINT('Ctrl Pts',(75.2379978491272,5.41211696232847,76.9218832987225));
#181501=CARTESIAN_POINT('Ctrl Pts',(75.2620568894032,5.4164426411786,76.9170539110535));
#181502=CARTESIAN_POINT('Ctrl Pts',(75.2383357398202,5.41644264187749,76.7825245638573));
#181503=CARTESIAN_POINT('Ctrl Pts',(75.2121521933087,5.41173498888793,76.7877804051212));
#181504=CARTESIAN_POINT('Ctrl Pts',(75.1860020711149,5.40682999840865,76.7930233592625));
#181505=CARTESIAN_POINT('Ctrl Pts',(75.1024038764153,5.39049755800644,76.8097669147133));
#181506=CARTESIAN_POINT('Ctrl Pts',(75.0450984412981,5.37831386775064,76.8212180196962));
#181507=CARTESIAN_POINT('Ctrl Pts',(74.7415135912732,5.3084979358921,76.8817824744488));
#181508=CARTESIAN_POINT('Ctrl Pts',(74.4991796415597,5.2342303228491,76.9297908415526));
#181509=CARTESIAN_POINT('Ctrl Pts',(74.018956833578,5.04867940242845,77.0252976914753));
#181510=CARTESIAN_POINT('Ctrl Pts',(73.7821034336695,4.93652837570146,77.0726083068148));
#181511=CARTESIAN_POINT('Ctrl Pts',(73.4744025257356,4.7621007935674,77.1348164042042));
#181512=CARTESIAN_POINT('Ctrl Pts',(73.3957235924925,4.71478566949915,77.1507910210769));
#181513=CARTESIAN_POINT('Ctrl Pts',(73.2580036214972,4.62706724569614,77.1788875048521));
#181514=CARTESIAN_POINT('Ctrl Pts',(73.1984912924057,4.58746739010145,77.1910751414921));
#181515=CARTESIAN_POINT('Ctrl Pts',(73.0694694418116,4.49784470077418,77.2176038127324));
#181516=CARTESIAN_POINT('Ctrl Pts',(73.0003220028763,4.4473194661203,77.2318916857073));
#181517=CARTESIAN_POINT('Ctrl Pts',(72.7579862368154,4.26120605798702,77.2822166701101));
#181518=CARTESIAN_POINT('Ctrl Pts',(72.591804339521,4.1165748527632,77.3172095753566));
#181519=CARTESIAN_POINT('Ctrl Pts',(72.2560280777784,3.78623421995547,77.3887529344337));
#181520=CARTESIAN_POINT('Ctrl Pts',(72.0895177288582,3.59800189436022,77.4247702123249));
#181521=CARTESIAN_POINT('Ctrl Pts',(71.8941598829739,3.34382649608401,77.467293904684));
#181522=CARTESIAN_POINT('Ctrl Pts',(71.8530114834805,3.28813581640704,77.4762668156286));
#181523=CARTESIAN_POINT('Ctrl Pts',(71.7883621853077,3.19708372001615,77.4903748302629));
#181524=CARTESIAN_POINT('Ctrl Pts',(71.7642079502864,3.16221692451688,77.4956480612288));
#181525=CARTESIAN_POINT('Ctrl Pts',(71.711584544796,3.08434613997645,77.5071381125684));
#181526=CARTESIAN_POINT('Ctrl Pts',(71.6833093419003,3.04121116067894,77.5133140609048));
#181527=CARTESIAN_POINT('Ctrl Pts',(71.589852058798,2.89417158313358,77.5337520085294));
#181528=CARTESIAN_POINT('Ctrl Pts',(71.5274994425849,2.78843289923142,77.547430623301));
#181529=CARTESIAN_POINT('Ctrl Pts',(71.3450888938553,2.45404469313372,77.5877832333549));
#181530=CARTESIAN_POINT('Ctrl Pts',(71.237397826488,2.21878568298582,77.612128993392));
#181531=CARTESIAN_POINT('Ctrl Pts',(71.1080121568317,1.8740638942293,77.6428669571353));
#181532=CARTESIAN_POINT('Ctrl Pts',(71.0725614609184,1.77034848667076,77.6515083564749));
#181533=CARTESIAN_POINT('Ctrl Pts',(71.01234594322,1.57544236173901,77.6666693743536));
#181534=CARTESIAN_POINT('Ctrl Pts',(70.986790834954,1.48454867398283,77.6733142641214));
#181535=CARTESIAN_POINT('Ctrl Pts',(70.9457537174226,1.32283159845772,77.6844058694877));
#181536=CARTESIAN_POINT('Ctrl Pts',(70.9293163151625,1.25228498081761,77.6890027211672));
#181537=CARTESIAN_POINT('Ctrl Pts',(70.8964622778505,1.09763050748786,77.6985595523389));
#181538=CARTESIAN_POINT('Ctrl Pts',(70.8806014113748,1.01341870140014,77.7034314598606));
#181539=CARTESIAN_POINT('Ctrl Pts',(70.8378257514775,0.753343661745575,
77.7174630723712));
#181540=CARTESIAN_POINT('Ctrl Pts',(70.8173962056347,0.576477258031514,
77.7255938220399));
#181541=CARTESIAN_POINT('Ctrl Pts',(70.7877817867805,0.135522831024074,
77.7422923261319));
#181542=CARTESIAN_POINT('Ctrl Pts',(70.7888313221881,-0.128868983708147,
77.749163479209));
#181543=CARTESIAN_POINT('Ctrl Pts',(70.8179937594841,-0.518410544724735,
77.7541583840847));
#181544=CARTESIAN_POINT('Ctrl Pts',(70.8317133884968,-0.644228455132306,
77.7549692474054));
#181545=CARTESIAN_POINT('Ctrl Pts',(70.8566253349969,-0.817951762691666,
77.7548966361948));
#181546=CARTESIAN_POINT('Ctrl Pts',(70.8642111310004,-0.866335518835818,
77.7547469582022));
#181547=CARTESIAN_POINT('Ctrl Pts',(70.8789446777879,-0.952896077184336,
77.7542402835623));
#181548=CARTESIAN_POINT('Ctrl Pts',(70.8858572987662,-0.99110887256114,
77.7539320561222));
#181549=CARTESIAN_POINT('Ctrl Pts',(70.9040476538424,-1.08603293809349,
77.7529580365788));
#181550=CARTESIAN_POINT('Ctrl Pts',(70.915805846609,-1.14264588965931,77.7521918835438));
#181551=CARTESIAN_POINT('Ctrl Pts',(70.9966400809492,-1.50369803834474,
77.7461599782457));
#181552=CARTESIAN_POINT('Ctrl Pts',(71.0901531602512,-1.80199378840545,
77.7359688303058));
#181553=CARTESIAN_POINT('Ctrl Pts',(71.294814503612,-2.30290023895625,77.7111391720313));
#181554=CARTESIAN_POINT('Ctrl Pts',(71.3945097168636,-2.50941346181454,
77.6984149052664));
#181555=CARTESIAN_POINT('Ctrl Pts',(71.5496997562606,-2.78567500115383,
77.6781214950324));
#181556=CARTESIAN_POINT('Ctrl Pts',(71.5945543093198,-2.86124526161526,
77.6722085006193));
#181557=CARTESIAN_POINT('Ctrl Pts',(71.6795377149533,-2.99694033929104,
77.6609314004789));
#181558=CARTESIAN_POINT('Ctrl Pts',(71.7190846943736,-3.05741330551257,
77.6556570891415));
#181559=CARTESIAN_POINT('Ctrl Pts',(71.8113305673564,-3.19259728148929,
77.6432984916175));
#181560=CARTESIAN_POINT('Ctrl Pts',(71.8647181737838,-3.26680234942626,
77.6361076342326));
#181561=CARTESIAN_POINT('Ctrl Pts',(72.0849079142146,-3.55732360316079,
77.6062963075679));
#181562=CARTESIAN_POINT('Ctrl Pts',(72.2657482708563,-3.76227939437997,
77.5815024458824));
#181563=CARTESIAN_POINT('Ctrl Pts',(72.5667355642835,-4.05613328083324,
77.5394092855849));
#181564=CARTESIAN_POINT('Ctrl Pts',(72.6766765676104,-4.15511079295192,
77.5238822408153));
#181565=CARTESIAN_POINT('Ctrl Pts',(72.842297519081,-4.29251415957608,77.500168283517));
#181566=CARTESIAN_POINT('Ctrl Pts',(72.8949550200511,-4.33458406741912,
77.4925837229831));
#181567=CARTESIAN_POINT('Ctrl Pts',(72.9925448899275,-4.4096444188691,77.47843061017));
#181568=CARTESIAN_POINT('Ctrl Pts',(73.0372356872186,-4.4429440650664,77.4719135345937));
#181569=CARTESIAN_POINT('Ctrl Pts',(73.116280046932,-4.49998457155734,77.460315802271));
#181570=CARTESIAN_POINT('Ctrl Pts',(73.15041497695,-4.5240277274252,77.4552840918951));
#181571=CARTESIAN_POINT('Ctrl Pts',(73.2275322192475,-4.57703449428552,
77.4438667000694));
#181572=CARTESIAN_POINT('Ctrl Pts',(73.270653839837,-4.60577930332613,77.4374492249423));
#181573=CARTESIAN_POINT('Ctrl Pts',(73.4392280095897,-4.71471384940827,
77.4122536502627));
#181574=CARTESIAN_POINT('Ctrl Pts',(73.5674688040901,-4.79032344700966,
77.392859769059));
#181575=CARTESIAN_POINT('Ctrl Pts',(73.9003579009783,-4.96858524161559,
77.3422318222505));
#181576=CARTESIAN_POINT('Ctrl Pts',(74.1086129192137,-5.06367883902265,
77.310306566457));
#181577=CARTESIAN_POINT('Ctrl Pts',(74.4194043542642,-5.18239691820562,
77.2627355876975));
#181578=CARTESIAN_POINT('Ctrl Pts',(74.5176759813545,-5.21671295687675,
77.2477020090433));
#181579=CARTESIAN_POINT('Ctrl Pts',(74.7035470299226,-5.27564158540855,
77.2193160764269));
#181580=CARTESIAN_POINT('Ctrl Pts',(74.79090048902,-5.30092267401602,77.2059951253706));
#181581=CARTESIAN_POINT('Ctrl Pts',(74.9481748430708,-5.34215609552141,
77.1820597763068));
#181582=CARTESIAN_POINT('Ctrl Pts',(75.0178572037227,-5.35894632324996,
77.1714714752744));
#181583=CARTESIAN_POINT('Ctrl Pts',(75.1727593487285,-5.39301436110121,
77.1479746126819));
#181584=CARTESIAN_POINT('Ctrl Pts',(75.2581029384633,-5.40962850005149,
77.1350559930417));
#181585=CARTESIAN_POINT('Ctrl Pts',(75.5525379293687,-5.45957942654126,
77.0905799650977));
#181586=CARTESIAN_POINT('Ctrl Pts',(75.763158296969,-5.48264371527299,77.0589329916905));
#181587=CARTESIAN_POINT('Ctrl Pts',(76.2031083107582,-5.50470442258212,
76.9930053001465));
#181588=CARTESIAN_POINT('Ctrl Pts',(76.4321381119054,-5.50158111730431,
76.9587842793382));
#181589=CARTESIAN_POINT('Ctrl Pts',(76.7778117505877,-5.47478068866244,
76.9069064286742));
#181590=CARTESIAN_POINT('Ctrl Pts',(76.8950284368944,-5.46180750578279,
76.8892722822737));
#181591=CARTESIAN_POINT('Ctrl Pts',(77.0588441352381,-5.43820561287079,
76.8645012484794));
#181592=CARTESIAN_POINT('Ctrl Pts',(77.1058745110634,-5.43079127042049,
76.8573748042622));
#181593=CARTESIAN_POINT('Ctrl Pts',(77.1907922217253,-5.41624621809818,
76.8444741869013));
#181594=CARTESIAN_POINT('Ctrl Pts',(77.2287123172768,-5.4093307798965,76.8387007532665));
#181595=CARTESIAN_POINT('Ctrl Pts',(77.3240446776781,-5.39088435093823,
76.8241573179166));
#181596=CARTESIAN_POINT('Ctrl Pts',(77.3813491211584,-5.37882236830412,
76.8153894297389));
#181597=CARTESIAN_POINT('Ctrl Pts',(77.7316389432862,-5.29909788155163,
76.7616802485711));
#181598=CARTESIAN_POINT('Ctrl Pts',(78.0187853615487,-5.20789914584257,
76.7171931143448));
#181599=CARTESIAN_POINT('Ctrl Pts',(78.5112659258398,-5.00485783530604,
76.6415294713727));
#181600=CARTESIAN_POINT('Ctrl Pts',(78.7196983601689,-4.90282012808141,
76.6097211452971));
#181601=CARTESIAN_POINT('Ctrl Pts',(78.9971787737498,-4.74421036598674,
76.5679696080069));
#181602=CARTESIAN_POINT('Ctrl Pts',(79.0721774994365,-4.69890366171995,
76.5567467104564));
#181603=CARTESIAN_POINT('Ctrl Pts',(79.2066784165441,-4.61315623753092,
76.5367433574633));
#181604=CARTESIAN_POINT('Ctrl Pts',(79.2665276897541,-4.57331508060458,
76.5278886651764));
#181605=CARTESIAN_POINT('Ctrl Pts',(79.4000994295692,-4.48053721038469,
76.5082350430473));
#181606=CARTESIAN_POINT('Ctrl Pts',(79.4733346747886,-4.42691566143916,
76.4975366348576));
#181607=CARTESIAN_POINT('Ctrl Pts',(79.7674343965113,-4.20012295502978,
76.4548894379693));
#181608=CARTESIAN_POINT('Ctrl Pts',(79.9763759104936,-4.01174434706531,
76.4253680399994));
#181609=CARTESIAN_POINT('Ctrl Pts',(80.312547334382,-3.65830305259652,76.3788158169302));
#181610=CARTESIAN_POINT('Ctrl Pts',(80.4464875160721,-3.50057980144184,
76.3605768787784));
#181611=CARTESIAN_POINT('Ctrl Pts',(80.6054013897789,-3.29050908060458,
76.3390749291356));
#181612=CARTESIAN_POINT('Ctrl Pts',(80.6388208439128,-3.24488689350982,
76.3345613056508));
#181613=CARTESIAN_POINT('Ctrl Pts',(80.6957620322285,-3.1645856415478,76.3268759964784));
#181614=CARTESIAN_POINT('Ctrl Pts',(80.7195993186736,-3.1301422246151,76.3236596437455));
#181615=CARTESIAN_POINT('Ctrl Pts',(80.7718628968255,-3.05275144795981,
76.316611529833));
#181616=CARTESIAN_POINT('Ctrl Pts',(80.8000851405014,-3.00966984574559,
76.3128089705924));
#181617=CARTESIAN_POINT('Ctrl Pts',(80.9723565348599,-2.73848186189781,
76.2896498998373));
#181618=CARTESIAN_POINT('Ctrl Pts',(81.100202013198,-2.50032034648427,76.2727143209912));
#181619=CARTESIAN_POINT('Ctrl Pts',(81.2985503851231,-2.05591375978791,
76.2480088434532));
#181620=CARTESIAN_POINT('Ctrl Pts',(81.3752213309863,-1.85310640980372,
76.2391066952939));
#181621=CARTESIAN_POINT('Ctrl Pts',(81.4674153817168,-1.55849397041057,
76.2297273589077));
#181622=CARTESIAN_POINT('Ctrl Pts',(81.4927199099784,-1.47002736294592,
76.2273501434604));
#181623=CARTESIAN_POINT('Ctrl Pts',(81.5340308173649,-1.3108550459338,76.2238651703388));
#181624=CARTESIAN_POINT('Ctrl Pts',(81.5508659261796,-1.2403906198054,76.222595204656));
#181625=CARTESIAN_POINT('Ctrl Pts',(81.5850645110894,-1.08387228916386,
76.2203786905601));
#181626=CARTESIAN_POINT('Ctrl Pts',(81.6017818015406,-0.99769577303986,
76.2195577540585));
#181627=CARTESIAN_POINT('Ctrl Pts',(81.6479195926949,-0.725831036467185,
76.2182171837524));
#181628=CARTESIAN_POINT('Ctrl Pts',(81.6700247373493,-0.539032751148363,
76.2191168628233));
#181629=CARTESIAN_POINT('Ctrl Pts',(81.6996439911372,-0.1004184491931,76.2253393397779));
#181630=CARTESIAN_POINT('Ctrl Pts',(81.6996422416693,0.151466148174329,
76.2320565924228));
#181631=CARTESIAN_POINT('Ctrl Pts',(81.6742570886569,0.525901404841964,
76.2462693347977));
#181632=CARTESIAN_POINT('Ctrl Pts',(81.6617677500643,0.649080374668952,
76.2516309395885));
#181633=CARTESIAN_POINT('Ctrl Pts',(81.6386551601267,0.819894052676462,
76.2599523369802));
#181634=CARTESIAN_POINT('Ctrl Pts',(81.6315027187836,0.86798682132388,76.2623938315713));
#181635=CARTESIAN_POINT('Ctrl Pts',(81.6175023714575,0.954300350311613,
76.2669471105319));
#181636=CARTESIAN_POINT('Ctrl Pts',(81.6108835537444,0.992555762755746,
76.2690255334203));
#181637=CARTESIAN_POINT('Ctrl Pts',(81.5933384536794,1.08797908170858,76.2743636544716));
#181638=CARTESIAN_POINT('Ctrl Pts',(81.5819129050912,1.14504590945925,76.2776953201407));
#181639=CARTESIAN_POINT('Ctrl Pts',(81.5041935953292,1.50378100727494,76.2995640680046));
#181640=CARTESIAN_POINT('Ctrl Pts',(81.4137245164432,1.79941399668105,76.3217616414451));
#181641=CARTESIAN_POINT('Ctrl Pts',(81.2138632637073,2.29937308767846,76.3682314719863));
#181642=CARTESIAN_POINT('Ctrl Pts',(81.1152788842141,2.50734621611064,76.3904997446754));
#181643=CARTESIAN_POINT('Ctrl Pts',(80.9617550773446,2.78506257271953,76.4246767954518));
#181644=CARTESIAN_POINT('Ctrl Pts',(80.9175467239182,2.86071612019881,76.4344698593547));
#181645=CARTESIAN_POINT('Ctrl Pts',(80.8337984729699,2.99649370119639,76.4529464558072));
#181646=CARTESIAN_POINT('Ctrl Pts',(80.7948398271277,3.05696817881084,76.4615146114001));
#181647=CARTESIAN_POINT('Ctrl Pts',(80.7040035991729,3.19207134774167,76.4814354468358));
#181648=CARTESIAN_POINT('Ctrl Pts',(80.6514465144278,3.26619715537172,76.4929227184661));
#181649=CARTESIAN_POINT('Ctrl Pts',(80.4325587421269,3.55919652385153,76.5406075062608));
#181650=CARTESIAN_POINT('Ctrl Pts',(80.2519225397787,3.76640761543606,76.5796380533348));
#181651=CARTESIAN_POINT('Ctrl Pts',(79.9109054377401,4.10248313616084,76.6523450992438));
#181652=CARTESIAN_POINT('Ctrl Pts',(79.7572470283821,4.23763541335688,76.684809279144));
#181653=CARTESIAN_POINT('Ctrl Pts',(79.5505286470775,4.39956203760259,76.7278397659946));
#181654=CARTESIAN_POINT('Ctrl Pts',(79.5040742195071,4.43474706847252,76.7374702657068));
#181655=CARTESIAN_POINT('Ctrl Pts',(79.4236840042652,4.49360083442434,76.7540588173398));
#181656=CARTESIAN_POINT('Ctrl Pts',(79.3900262930399,4.51764875494748,76.7609809584647));
#181657=CARTESIAN_POINT('Ctrl Pts',(79.3081665181275,4.57471749697913,76.7777616449163));
#181658=CARTESIAN_POINT('Ctrl Pts',(79.2597018907612,4.60734063210637,76.7876528358797));
#181659=CARTESIAN_POINT('Ctrl Pts',(79.0201606754448,4.76295692565485,76.8363659483317));
#181660=CARTESIAN_POINT('Ctrl Pts',(78.822064602832,4.87441600835014,76.8761231658563));
#181661=CARTESIAN_POINT('Ctrl Pts',(78.4601385650249,5.04876078011816,76.9485274962522));
#181662=CARTESIAN_POINT('Ctrl Pts',(78.299080659993,5.11682025036021,76.9806703048635));
#181663=CARTESIAN_POINT('Ctrl Pts',(78.0173195421672,5.21989599301449,77.036977655885));
#181664=CARTESIAN_POINT('Ctrl Pts',(77.8981260804415,5.25878695607624,77.0608186087014));
#181665=CARTESIAN_POINT('Ctrl Pts',(77.7053427287116,5.31423596032044,77.099455942848));
#181666=CARTESIAN_POINT('Ctrl Pts',(77.6325461967876,5.33350858403807,77.1140626305387));
#181667=CARTESIAN_POINT('Ctrl Pts',(77.4870824509904,5.36872788955947,77.1432899705638));
#181668=CARTESIAN_POINT('Ctrl Pts',(77.4144396234916,5.38470734859668,77.157905251409));
#181669=CARTESIAN_POINT('Ctrl Pts',(77.2259253519114,5.42203777861132,77.1958863954788));
#181670=CARTESIAN_POINT('Ctrl Pts',(77.1096571961192,5.44105857751182,77.2193637990583));
#181671=CARTESIAN_POINT('Ctrl Pts',(76.6568029097262,5.49971206463977,77.3109870896955));
#181672=CARTESIAN_POINT('Ctrl Pts',(76.3175287645782,5.51084061050336,77.3800709114985));
#181673=CARTESIAN_POINT('Ctrl Pts',(75.8422763109589,5.48073681899623,77.4765294975149));
#181674=CARTESIAN_POINT('Ctrl Pts',(75.7054604318992,5.46669980131952,77.5042523148631));
#181675=CARTESIAN_POINT('Ctrl Pts',(75.5204176104763,5.44039768868911,77.5415814812565));
#181676=CARTESIAN_POINT('Ctrl Pts',(75.4716301663453,5.4327658233183,77.551407556646));
#181677=CARTESIAN_POINT('Ctrl Pts',(75.4077060172307,5.42184898014661,77.5642560808688));
#181678=CARTESIAN_POINT('Ctrl Pts',(75.3924745342712,5.41917915681955,77.5673155945721));
#181679=CARTESIAN_POINT('Ctrl Pts',(75.3772542827084,5.41644264201317,77.5703707661157));
#181680=CARTESIAN_POINT('Origin',(76.0518331668413,7.15881389286582E-15,
75.8960977421633));
#181681=CARTESIAN_POINT('',(75.5398939750202,5.41644264142069,78.4927463156221));
#181682=CARTESIAN_POINT('',(75.5161728235182,5.41644264177605,78.3582169687627));
#181683=CARTESIAN_POINT('',(75.1112777726958,5.41644264156718,76.061943035002));
#181684=CARTESIAN_POINT('Ctrl Pts',(75.539893974202,5.41644264127421,78.4927463157663));
#181685=CARTESIAN_POINT('Ctrl Pts',(75.5665177744018,5.42122944939478,78.4874021020774));
#181686=CARTESIAN_POINT('Ctrl Pts',(75.5931778794221,5.42581209806781,78.4820587179476));
#181687=CARTESIAN_POINT('Ctrl Pts',(75.6780941552782,5.43973924578088,78.4650625654341));
#181688=CARTESIAN_POINT('Ctrl Pts',(75.736472255955,5.44831432884837,78.4534128479944));
#181689=CARTESIAN_POINT('Ctrl Pts',(76.0388879342549,5.48758406675844,78.3932023552001));
#181690=CARTESIAN_POINT('Ctrl Pts',(76.2847154158278,5.50222399328912,78.3447107407262));
#181691=CARTESIAN_POINT('Ctrl Pts',(76.8039561365274,5.49695258744133,78.2422088614041));
#181692=CARTESIAN_POINT('Ctrl Pts',(77.0766369260728,5.47302616476621,78.1883248440585));
#181693=CARTESIAN_POINT('Ctrl Pts',(77.4341038940642,5.41354181212434,78.1170945890549));
#181694=CARTESIAN_POINT('Ctrl Pts',(77.5215466371534,5.39671587684082,78.099625106959));
#181695=CARTESIAN_POINT('Ctrl Pts',(77.6779665538692,5.36250843993205,78.0682829388475));
#181696=CARTESIAN_POINT('Ctrl Pts',(77.7470943070347,5.345927359775,78.0543988745758));
#181697=CARTESIAN_POINT('Ctrl Pts',(77.9002886642604,5.3059077551178,78.0235543818294));
#181698=CARTESIAN_POINT('Ctrl Pts',(77.9841565591565,5.28177314589311,78.0066165093496));
#181699=CARTESIAN_POINT('Ctrl Pts',(78.3605939814393,5.16331813944078,77.9303615599141));
#181700=CARTESIAN_POINT('Ctrl Pts',(78.6454063153438,5.04570520662327,77.8719908223492));
#181701=CARTESIAN_POINT('Ctrl Pts',(79.0316094029643,4.84556850245134,77.7924229256697));
#181702=CARTESIAN_POINT('Ctrl Pts',(79.1423525774821,4.783076466589,77.7695608083373));
#181703=CARTESIAN_POINT('Ctrl Pts',(79.3233867615088,4.67225345573668,77.7321965985497));
#181704=CARTESIAN_POINT('Ctrl Pts',(79.3949004820337,4.62610461423978,77.7174393964842));
#181705=CARTESIAN_POINT('Ctrl Pts',(79.5021780677057,4.55321638765529,77.6953345547157));
#181706=CARTESIAN_POINT('Ctrl Pts',(79.5387295261656,4.52771378140688,77.6878089896472));
#181707=CARTESIAN_POINT('Ctrl Pts',(79.6126288791184,4.47477958502922,77.6726118823387));
#181708=CARTESIAN_POINT('Ctrl Pts',(79.6499487686035,4.44731388034164,77.6649465238731));
#181709=CARTESIAN_POINT('Ctrl Pts',(79.763857294428,4.36120081958458,77.6415675260766));
#181710=CARTESIAN_POINT('Ctrl Pts',(79.8392665766835,4.3009554250436,77.6261146969504));
#181711=CARTESIAN_POINT('Ctrl Pts',(80.0885517739142,4.09062617508746,77.575007143717));
#181712=CARTESIAN_POINT('Ctrl Pts',(80.2546623615278,3.93136059134858,77.540901272547));
#181713=CARTESIAN_POINT('Ctrl Pts',(80.5469721753666,3.6130712372858,77.4801270270181));
#181714=CARTESIAN_POINT('Ctrl Pts',(80.675338443127,3.45664993780459,77.4531076505331));
#181715=CARTESIAN_POINT('Ctrl Pts',(80.8446335728154,3.22520743598249,77.4167701536957));
#181716=CARTESIAN_POINT('Ctrl Pts',(80.8928821644023,3.15593243815639,77.4063225217695));
#181717=CARTESIAN_POINT('Ctrl Pts',(80.9793699369941,3.02540562892804,77.3874092379275));
#181718=CARTESIAN_POINT('Ctrl Pts',(81.0180347572513,2.96446807389958,77.3788784977968));
#181719=CARTESIAN_POINT('Ctrl Pts',(81.103945991764,2.82295789762348,77.3597415211337));
#181720=CARTESIAN_POINT('Ctrl Pts',(81.1503673026584,2.74189385766077,77.34926377095));
#181721=CARTESIAN_POINT('Ctrl Pts',(81.3389322659218,2.39219405932335,77.3060957666568));
#181722=CARTESIAN_POINT('Ctrl Pts',(81.4608682045296,2.1128937399139,77.2765636093171));
#181723=CARTESIAN_POINT('Ctrl Pts',(81.6291238048297,1.62027344458349,77.2331341000539));
#181724=CARTESIAN_POINT('Ctrl Pts',(81.6869793911751,1.41182088629801,77.2172364300291));
#181725=CARTESIAN_POINT('Ctrl Pts',(81.744848212222,1.14376142834612,77.2001896136743));
#181726=CARTESIAN_POINT('Ctrl Pts',(81.756193292366,1.08693827933067,77.196766004603));
#181727=CARTESIAN_POINT('Ctrl Pts',(81.7736595126025,0.991782815014574,
77.1913585623123));
#181728=CARTESIAN_POINT('Ctrl Pts',(81.780267274009,0.95355062558589,77.1892733976972));
#181729=CARTESIAN_POINT('Ctrl Pts',(81.7942845049315,0.867106454502926,
77.1847574348103));
#181730=CARTESIAN_POINT('Ctrl Pts',(81.8014629076115,0.818858855285828,
77.1823747812565));
#181731=CARTESIAN_POINT('Ctrl Pts',(81.8232991949716,0.657647323237761,
77.1748585102432));
#181732=CARTESIAN_POINT('Ctrl Pts',(81.8351448082689,0.544306046995467,
77.1702997685963));
#181733=CARTESIAN_POINT('Ctrl Pts',(81.8601302274017,0.205323124238502,
77.1586740364029));
#181734=CARTESIAN_POINT('Ctrl Pts',(81.8630760930305,-0.0208904111426021,
77.153548546791));
#181735=CARTESIAN_POINT('Ctrl Pts',(81.8416333136685,-0.469678367629121,
77.1479806705861));
#181736=CARTESIAN_POINT('Ctrl Pts',(81.8176059884919,-0.691840792123546,
77.1474843552474));
#181737=CARTESIAN_POINT('Ctrl Pts',(81.7656605759851,-0.998399353691106,
77.1497162701339));
#181738=CARTESIAN_POINT('Ctrl Pts',(81.7489733665241,-1.08448547846655,
77.1506705045438));
#181739=CARTESIAN_POINT('Ctrl Pts',(81.7147973777085,-1.24091561850257,
77.1529962619806));
#181740=CARTESIAN_POINT('Ctrl Pts',(81.6979543901176,-1.31138186176718,
77.1542663758805));
#181741=CARTESIAN_POINT('Ctrl Pts',(81.6565793458909,-1.47065992964979,
77.1576425557935));
#181742=CARTESIAN_POINT('Ctrl Pts',(81.6312081541514,-1.55922839791175,
77.1598813253126));
#181743=CARTESIAN_POINT('Ctrl Pts',(81.5251334061915,-1.89754847118375,
77.1698397729302));
#181744=CARTESIAN_POINT('Ctrl Pts',(81.4290088648005,-2.14202658181963,
77.1800073105019));
#181745=CARTESIAN_POINT('Ctrl Pts',(81.2178244812093,-2.58447503603234,
77.2044962166762));
#181746=CARTESIAN_POINT('Ctrl Pts',(81.107078627218,-2.78391628561171,77.2180846176862));
#181747=CARTESIAN_POINT('Ctrl Pts',(80.9547211756227,-3.02249305235994,
77.23796019709));
#181748=CARTESIAN_POINT('Ctrl Pts',(80.9242504733597,-3.06867106612347,
77.2419864274865));
#181749=CARTESIAN_POINT('Ctrl Pts',(80.8694518813549,-3.14907872777962,
77.2493242229635));
#181750=CARTESIAN_POINT('Ctrl Pts',(80.8454142331833,-3.18350427181685,
77.2525748156828));
#181751=CARTESIAN_POINT('Ctrl Pts',(80.7903402315579,-3.26050184647792,
77.2600907351692));
#181752=CARTESIAN_POINT('Ctrl Pts',(80.759086106593,-3.30290706193398,77.2644021846048));
#181753=CARTESIAN_POINT('Ctrl Pts',(80.5529060598978,-3.57444877781847,
77.2931039888029));
#181754=CARTESIAN_POINT('Ctrl Pts',(80.3610916192709,-3.78981818478707,
77.3209626744609));
#181755=CARTESIAN_POINT('Ctrl Pts',(80.032894428121,-4.10457922742631,77.3691737981482));
#181756=CARTESIAN_POINT('Ctrl Pts',(79.9071760571658,-4.21456305559467,
77.3877536693471));
#181757=CARTESIAN_POINT('Ctrl Pts',(79.6964759482369,-4.3824785826316,77.4189258860813));
#181758=CARTESIAN_POINT('Ctrl Pts',(79.6145099103994,-4.4441013151181,77.4310606536501));
#181759=CARTESIAN_POINT('Ctrl Pts',(79.4714425315016,-4.5454659874014,77.4522343788641));
#181760=CARTESIAN_POINT('Ctrl Pts',(79.4111810034324,-4.58636957987044,
77.4611511255962));
#181761=CARTESIAN_POINT('Ctrl Pts',(79.2824435024045,-4.67002469736474,
77.4801913097735));
#181762=CARTESIAN_POINT('Ctrl Pts',(79.2138022409961,-4.7124840117394,77.4903382116346));
#181763=CARTESIAN_POINT('Ctrl Pts',(79.0088055627473,-4.8330554741738,77.520624817344));
#181764=CARTESIAN_POINT('Ctrl Pts',(78.8700136197773,-4.90677137793196,
77.5411063367843));
#181765=CARTESIAN_POINT('Ctrl Pts',(78.4666325986895,-5.09903904193516,
77.6006293258309));
#181766=CARTESIAN_POINT('Ctrl Pts',(78.19557530012,-5.2024695344964,77.6406004346359));
#181767=CARTESIAN_POINT('Ctrl Pts',(77.7923905848181,-5.32027052228391,
77.7006639132548));
#181768=CARTESIAN_POINT('Ctrl Pts',(77.6657863908134,-5.35232805272204,
77.7196129603252));
#181769=CARTESIAN_POINT('Ctrl Pts',(77.4902721291951,-5.39005450177877,
77.7460901716236));
#181770=CARTESIAN_POINT('Ctrl Pts',(77.4422228882026,-5.39969944360075,
77.7533598907504));
#181771=CARTESIAN_POINT('Ctrl Pts',(77.356371468833,-5.41571833554547,77.7663934223048));
#181772=CARTESIAN_POINT('Ctrl Pts',(77.3186187131513,-5.42234669763438,
77.7721406762334));
#181773=CARTESIAN_POINT('Ctrl Pts',(77.2252250163596,-5.4377188694759,77.7863951795287));
#181774=CARTESIAN_POINT('Ctrl Pts',(77.1695160911954,-5.44599317496177,
77.7949292800279));
#181775=CARTESIAN_POINT('Ctrl Pts',(76.8372154834731,-5.49003172615719,
77.8459811802899));
#181776=CARTESIAN_POINT('Ctrl Pts',(76.5584531980336,-5.50510778397451,
77.8893903313261));
#181777=CARTESIAN_POINT('Ctrl Pts',(76.1083264897795,-5.49440722766906,
77.9593238512352));
#181778=CARTESIAN_POINT('Ctrl Pts',(75.9371778566939,-5.48212687548678,
77.9858810115573));
#181779=CARTESIAN_POINT('Ctrl Pts',(75.6408816836138,-5.44655971238055,
78.0316220270123));
#181780=CARTESIAN_POINT('Ctrl Pts',(75.5154466702457,-5.42698022544971,
78.0509127230922));
#181781=CARTESIAN_POINT('Ctrl Pts',(75.3159703938534,-5.38857655219032,
78.0814341344305));
#181782=CARTESIAN_POINT('Ctrl Pts',(75.2414546673423,-5.37258453259202,
78.0928005470773));
#181783=CARTESIAN_POINT('Ctrl Pts',(75.0946146671494,-5.33779886895718,
78.1151245375217));
#181784=CARTESIAN_POINT('Ctrl Pts',(75.0222922080519,-5.31907169105309,
78.1260833502294));
#181785=CARTESIAN_POINT('Ctrl Pts',(74.8368021017929,-5.26690931205343,
78.1540949802533));
#181786=CARTESIAN_POINT('Ctrl Pts',(74.7242785253933,-5.23124996817579,
78.1709945634405));
#181787=CARTESIAN_POINT('Ctrl Pts',(74.3398078049906,-5.09540708842723,
78.2284402534059));
#181788=CARTESIAN_POINT('Ctrl Pts',(74.0746000097748,-4.97701955461648,
78.2675163437505));
#181789=CARTESIAN_POINT('Ctrl Pts',(73.7313011908467,-4.78946040492022,
78.3178752737851));
#181790=CARTESIAN_POINT('Ctrl Pts',(73.6439977997442,-4.73855022028711,
78.3306644366919));
#181791=CARTESIAN_POINT('Ctrl Pts',(73.4955764613371,-4.64635541206792,
78.3524227783711));
#181792=CARTESIAN_POINT('Ctrl Pts',(73.4337933629486,-4.60621428909561,
78.3614851758109));
#181793=CARTESIAN_POINT('Ctrl Pts',(73.3372492650909,-4.54065805615898,
78.3756732415354));
#181794=CARTESIAN_POINT('Ctrl Pts',(73.3019473937524,-4.51606972317767,
78.3808672337088));
#181795=CARTESIAN_POINT('Ctrl Pts',(73.226402737355,-4.46210813065752,78.391999609484));
#181796=CARTESIAN_POINT('Ctrl Pts',(73.1862635163578,-4.43259519678838,
78.3979245779364));
#181797=CARTESIAN_POINT('Ctrl Pts',(73.0624666791677,-4.33892590448478,
78.4162155966171));
#181798=CARTESIAN_POINT('Ctrl Pts',(72.9802457930082,-4.27287452337565,
78.4283886038132));
#181799=CARTESIAN_POINT('Ctrl Pts',(72.6913081152475,-4.02664801642228,
78.4711133431972));
#181800=CARTESIAN_POINT('Ctrl Pts',(72.4961623461945,-3.8332272260895,78.4998475892305));
#181801=CARTESIAN_POINT('Ctrl Pts',(72.2427783739239,-3.54140578457545,
78.5362132391252));
#181802=CARTESIAN_POINT('Ctrl Pts',(72.1720308182705,-3.45473404833687,
78.5462495398058));
#181803=CARTESIAN_POINT('Ctrl Pts',(72.0457369173167,-3.29004489748573,
78.5638980712231));
#181804=CARTESIAN_POINT('Ctrl Pts',(71.9894974938757,-3.21262862070271,
78.5716476851331));
#181805=CARTESIAN_POINT('Ctrl Pts',(71.8942240416732,-3.07406705999987,
78.5845613453887));
#181806=CARTESIAN_POINT('Ctrl Pts',(71.8543389364359,-3.01355190715957,
78.5898949500262));
#181807=CARTESIAN_POINT('Ctrl Pts',(71.7704073344689,-2.8806106621182,78.6009522410751));
#181808=CARTESIAN_POINT('Ctrl Pts',(71.726807506194,-2.80791750331427,78.6065880412601));
#181809=CARTESIAN_POINT('Ctrl Pts',(71.6004339582427,-2.58585417145264,
78.6225838289649));
#181810=CARTESIAN_POINT('Ctrl Pts',(71.5228300266418,-2.43358973231042,
78.6319284667187));
#181811=CARTESIAN_POINT('Ctrl Pts',(71.3402112241093,-2.03044610650507,
78.652656119707));
#181812=CARTESIAN_POINT('Ctrl Pts',(71.2462903045331,-1.77494639163289,
78.6619469790285));
#181813=CARTESIAN_POINT('Ctrl Pts',(71.1361186458503,-1.39041840739252,
78.6709859916902));
#181814=CARTESIAN_POINT('Ctrl Pts',(71.1050972657586,-1.26610252129917,
78.6731835867271));
#181815=CARTESIAN_POINT('Ctrl Pts',(71.0681546925613,-1.09275858434809,
78.675333330361));
#181816=CARTESIAN_POINT('Ctrl Pts',(71.0585497610332,-1.04456345494294,
78.6758346158716));
#181817=CARTESIAN_POINT('Ctrl Pts',(71.0425063765194,-0.958089087027191,
78.676568349917));
#181818=CARTESIAN_POINT('Ctrl Pts',(71.0358274989382,-0.91985910316115,
78.6768357216557));
#181819=CARTESIAN_POINT('Ctrl Pts',(71.0202391821798,-0.824762928478273,
78.6773571363275));
#181820=CARTESIAN_POINT('Ctrl Pts',(71.0118118691523,-0.767822499697789,
78.6775415709439));
#181821=CARTESIAN_POINT('Ctrl Pts',(70.9631488273098,-0.399653947324125,
78.6778684629793));
#181822=CARTESIAN_POINT('Ctrl Pts',(70.9484260216193,-0.0856397834854804,
78.6741369816039));
#181823=CARTESIAN_POINT('Ctrl Pts',(70.968621281735,0.456166789450836,78.6593018635788));
#181824=CARTESIAN_POINT('Ctrl Pts',(70.9911209463974,0.68367151133436,78.650497229422));
#181825=CARTESIAN_POINT('Ctrl Pts',(71.0414320539691,0.995821165341956,
78.6345756643245));
#181826=CARTESIAN_POINT('Ctrl Pts',(71.057461944349,1.0822404374931,78.6297541703661));
#181827=CARTESIAN_POINT('Ctrl Pts',(71.0903831498529,1.23899471873172,78.6202425210799));
#181828=CARTESIAN_POINT('Ctrl Pts',(71.1066171634054,1.30945506728566,78.6156810242576));
#181829=CARTESIAN_POINT('Ctrl Pts',(71.1464951642544,1.46835047768269,78.6047409343273));
#181830=CARTESIAN_POINT('Ctrl Pts',(71.1709546760956,1.5565475755069,78.5982036220449));
#181831=CARTESIAN_POINT('Ctrl Pts',(71.2765333922488,1.90376887941866,78.5706167117745));
#181832=CARTESIAN_POINT('Ctrl Pts',(71.3743113914344,2.15706435303863,78.5463327671822));
#181833=CARTESIAN_POINT('Ctrl Pts',(71.5538605775691,2.53655989634403,78.503714009829));
#181834=CARTESIAN_POINT('Ctrl Pts',(71.6229752197624,2.66852330555532,78.4876395622037));
#181835=CARTESIAN_POINT('Ctrl Pts',(71.7311117628383,2.85602254511148,78.4630476428724));
#181836=CARTESIAN_POINT('Ctrl Pts',(71.7659744502709,2.91396650301486,78.4551933440778));
#181837=CARTESIAN_POINT('Ctrl Pts',(71.8315758297514,3.01856094504793,78.4405610247926));
#181838=CARTESIAN_POINT('Ctrl Pts',(71.8619763120377,3.06542003597401,78.4338336662169));
#181839=CARTESIAN_POINT('Ctrl Pts',(71.9163318417643,3.14645162855411,78.4219058391388));
#181840=CARTESIAN_POINT('Ctrl Pts',(71.9399722326786,3.18083431925575,78.4167503194992));
#181841=CARTESIAN_POINT('Ctrl Pts',(71.9937660405051,3.25718009657928,78.4050877751693));
#181842=CARTESIAN_POINT('Ctrl Pts',(72.0241234831559,3.29898860917227,78.3985518950606));
#181843=CARTESIAN_POINT('Ctrl Pts',(72.2297334469484,3.57385211125529,78.3545483118859));
#181844=CARTESIAN_POINT('Ctrl Pts',(72.42264726793,3.79267421678239,78.3144783538201));
#181845=CARTESIAN_POINT('Ctrl Pts',(72.7499304046403,4.10878341039927,78.2470501284729));
#181846=CARTESIAN_POINT('Ctrl Pts',(72.8730484526604,4.21733885557447,78.221793698017));
#181847=CARTESIAN_POINT('Ctrl Pts',(73.0799640708631,4.38370528203187,78.1793791948582));
#181848=CARTESIAN_POINT('Ctrl Pts',(73.1608731819593,4.44508420747317,78.1628022110368));
#181849=CARTESIAN_POINT('Ctrl Pts',(73.302254780683,4.54618307035463,78.133828427201));
#181850=CARTESIAN_POINT('Ctrl Pts',(73.3619072495882,4.58704970840229,78.1216017655663));
#181851=CARTESIAN_POINT('Ctrl Pts',(73.4894959199848,4.67073247008104,78.0954416852499));
#181852=CARTESIAN_POINT('Ctrl Pts',(73.5575996432741,4.71324952918654,78.0814729018663));
#181853=CARTESIAN_POINT('Ctrl Pts',(73.7616905816327,4.8343910698883,78.0395943951052));
#181854=CARTESIAN_POINT('Ctrl Pts',(73.900125837051,4.90854005609326,78.0111636560783));
#181855=CARTESIAN_POINT('Ctrl Pts',(74.2994943305779,5.10033784862872,77.929141629216));
#181856=CARTESIAN_POINT('Ctrl Pts',(74.5666851817975,5.20314329706973,77.8742417152858));
#181857=CARTESIAN_POINT('Ctrl Pts',(74.9269828464728,5.30934202677185,77.8007639257383));
#181858=CARTESIAN_POINT('Ctrl Pts',(75.0139270501562,5.33258114578658,77.7830763097766));
#181859=CARTESIAN_POINT('Ctrl Pts',(75.166994885496,5.36934406062368,77.7520488281465));
#181860=CARTESIAN_POINT('Ctrl Pts',(75.2328687744806,5.38384044302114,77.7387317678352));
#181861=CARTESIAN_POINT('Ctrl Pts',(75.3329277893673,5.40386335678467,77.7185726417664));
#181862=CARTESIAN_POINT('Ctrl Pts',(75.3669210508875,5.41031985689093,77.7117358726658));
#181863=CARTESIAN_POINT('Ctrl Pts',(75.4009754336941,5.41644264156649,77.7049001130302));
#181864=CARTESIAN_POINT('Ctrl Pts',(75.3772542827084,5.41644264201317,77.5703707661157));
#181865=CARTESIAN_POINT('Ctrl Pts',(75.3551306632751,5.41246494086284,77.5748116554304));
#181866=CARTESIAN_POINT('Ctrl Pts',(75.3330307739513,5.40834633171858,77.5792433706657));
#181867=CARTESIAN_POINT('Ctrl Pts',(75.2571593468384,5.39370708975354,77.5944443211266));
#181868=CARTESIAN_POINT('Ctrl Pts',(75.2035167710473,5.38249264657263,77.6051681275127));
#181869=CARTESIAN_POINT('Ctrl Pts',(74.8673311105018,5.30675913195313,77.6722670827772));
#181870=CARTESIAN_POINT('Ctrl Pts',(74.5900166783592,5.2199703866233,77.727155541709));
#181871=CARTESIAN_POINT('Ctrl Pts',(74.1681931649929,5.04902273212223,77.8111284089395));
#181872=CARTESIAN_POINT('Ctrl Pts',(74.0183340153448,4.98004591998959,77.8410578583084));
#181873=CARTESIAN_POINT('Ctrl Pts',(73.7619402997817,4.84731565757822,77.8925954191191));
#181874=CARTESIAN_POINT('Ctrl Pts',(73.6540142440242,4.78660439634999,77.9143977290939));
#181875=CARTESIAN_POINT('Ctrl Pts',(73.4837556395166,4.68289376102598,77.9490048065502));
#181876=CARTESIAN_POINT('Ctrl Pts',(73.4200865652762,4.64224053912069,77.9619961894697));
#181877=CARTESIAN_POINT('Ctrl Pts',(73.2951293503213,4.55868535663434,77.9875984063133));
#181878=CARTESIAN_POINT('Ctrl Pts',(73.2338368344033,4.51582034164073,78.0002090200944));
#181879=CARTESIAN_POINT('Ctrl Pts',(73.0766053921483,4.40089612641961,78.0326981335471));
#181880=CARTESIAN_POINT('Ctrl Pts',(72.9821200638585,4.3268594986081,78.0523623813962));
#181881=CARTESIAN_POINT('Ctrl Pts',(72.6694402219715,4.06452273194333,78.1178964355982));
#181882=CARTESIAN_POINT('Ctrl Pts',(72.4636574405655,3.86172294495375,78.1618513475365));
#181883=CARTESIAN_POINT('Ctrl Pts',(72.2099623126922,3.56839580079293,78.2166814682362));
#181884=CARTESIAN_POINT('Ctrl Pts',(72.1472678171828,3.49178931474804,78.230289047022));
#181885=CARTESIAN_POINT('Ctrl Pts',(72.0421899545113,3.35603549676313,78.2531540813623));
#181886=CARTESIAN_POINT('Ctrl Pts',(71.9988559849183,3.29768821002673,78.2626022152662));
#181887=CARTESIAN_POINT('Ctrl Pts',(71.9318111555133,3.20356605885862,78.2772320799985));
#181888=CARTESIAN_POINT('Ctrl Pts',(71.9073496634705,3.16836087057786,78.2825723246921));
#181889=CARTESIAN_POINT('Ctrl Pts',(71.8551700506616,3.09135817231146,78.2939651380305));
#181890=CARTESIAN_POINT('Ctrl Pts',(71.8276048236484,3.04945806195616,78.2999855424708));
#181891=CARTESIAN_POINT('Ctrl Pts',(71.7427282493247,2.91652037943227,78.3185437502732));
#181892=CARTESIAN_POINT('Ctrl Pts',(71.6874823286298,2.82413590909042,78.3306544083646));
#181893=CARTESIAN_POINT('Ctrl Pts',(71.5022572925732,2.49271866192628,78.371525469451));
#181894=CARTESIAN_POINT('Ctrl Pts',(71.3871468829608,2.24549796197737,78.3974526902117));
#181895=CARTESIAN_POINT('Ctrl Pts',(71.2640528520746,1.92020105936863,78.4266332599623));
#181896=CARTESIAN_POINT('Ctrl Pts',(71.2388690923248,1.8493134666371,78.4327052831731));
#181897=CARTESIAN_POINT('Ctrl Pts',(71.1797768411235,1.67156520371003,78.4472397172474));
#181898=CARTESIAN_POINT('Ctrl Pts',(71.1476474192826,1.56412638737289,78.4554139430176));
#181899=CARTESIAN_POINT('Ctrl Pts',(71.0996585460341,1.38388449494464,78.4681484903561));
#181900=CARTESIAN_POINT('Ctrl Pts',(71.0819693264505,1.31162489661964,78.4729970910972));
#181901=CARTESIAN_POINT('Ctrl Pts',(71.0486482107059,1.16258278093309,78.482479040289));
#181902=CARTESIAN_POINT('Ctrl Pts',(71.0331777364175,1.08577989366263,78.4870864964874));
#181903=CARTESIAN_POINT('Ctrl Pts',(70.99501289964,0.873149227891994,78.4990803089403));
#181904=CARTESIAN_POINT('Ctrl Pts',(70.9757320723611,0.736737432565285,
78.5059261166379));
#181905=CARTESIAN_POINT('Ctrl Pts',(70.9413112111456,0.404602046368871,
78.520524399549));
#181906=CARTESIAN_POINT('Ctrl Pts',(70.9314168130957,0.208487155890121,
78.5274236904707));
#181907=CARTESIAN_POINT('Ctrl Pts',(70.9324223884411,-0.224800901825671,
78.5386663569182));
#181908=CARTESIAN_POINT('Ctrl Pts',(70.9480635829902,-0.461601469887723,
78.5421726518326));
#181909=CARTESIAN_POINT('Ctrl Pts',(70.9863635500486,-0.756066219738908,
78.5428292352717));
#181910=CARTESIAN_POINT('Ctrl Pts',(70.9950334161317,-0.815295897793722,
78.5427708069543));
#181911=CARTESIAN_POINT('Ctrl Pts',(71.0109206396469,-0.912915291205025,
78.5423486093226));
#181912=CARTESIAN_POINT('Ctrl Pts',(71.0175946239952,-0.951388755684431,
78.5420978021178));
#181913=CARTESIAN_POINT('Ctrl Pts',(71.0333257423385,-1.0367778158736,78.5413509608545));
#181914=CARTESIAN_POINT('Ctrl Pts',(71.0425812932071,-1.08365230719983,
78.5408135609644));
#181915=CARTESIAN_POINT('Ctrl Pts',(71.0764055856693,-1.24413800401546,
78.5385484675323));
#181916=CARTESIAN_POINT('Ctrl Pts',(71.1039042681785,-1.35709090290732,
78.5362195797992));
#181917=CARTESIAN_POINT('Ctrl Pts',(71.1934290721886,-1.68059364153978,
78.5275635981392));
#181918=CARTESIAN_POINT('Ctrl Pts',(71.2643449283296,-1.88840066118407,
78.5195369611606));
#181919=CARTESIAN_POINT('Ctrl Pts',(71.4322724944426,-2.29924745081154,
78.4991612329898));
#181920=CARTESIAN_POINT('Ctrl Pts',(71.5297081509498,-2.50166271137656,
78.4867348914563));
#181921=CARTESIAN_POINT('Ctrl Pts',(71.6827111072875,-2.77556385226428,
78.4667446956249));
#181922=CARTESIAN_POINT('Ctrl Pts',(71.7281923492761,-2.85253694011235,
78.4607526491086));
#181923=CARTESIAN_POINT('Ctrl Pts',(71.8137575012774,-2.98963833760957,
78.4494031203047));
#181924=CARTESIAN_POINT('Ctrl Pts',(71.8531959219295,-3.05015323918425,
78.4441452894191));
#181925=CARTESIAN_POINT('Ctrl Pts',(71.9442722491566,-3.18407814421525,
78.4319477378013));
#181926=CARTESIAN_POINT('Ctrl Pts',(71.9965330672359,-3.25703049324408,
78.424911617405));
#181927=CARTESIAN_POINT('Ctrl Pts',(72.1987427780659,-3.52521697386439,
78.3975484236171));
#181928=CARTESIAN_POINT('Ctrl Pts',(72.3598588773342,-3.71148662420113,
78.3754908419883));
#181929=CARTESIAN_POINT('Ctrl Pts',(72.7028229027418,-4.05804666259696,
78.3277333828107));
#181930=CARTESIAN_POINT('Ctrl Pts',(72.8839141088621,-4.21833837794861,
78.302148057298));
#181931=CARTESIAN_POINT('Ctrl Pts',(73.1163156600455,-4.39815580145707,
78.2684790005611));
#181932=CARTESIAN_POINT('Ctrl Pts',(73.1582928590878,-4.429680255181,78.2623662342311));
#181933=CARTESIAN_POINT('Ctrl Pts',(73.2345053836241,-4.48521880950411,
78.2512045193478));
#181934=CARTESIAN_POINT('Ctrl Pts',(73.2685780405339,-4.50945549544521,
78.2461917010365));
#181935=CARTESIAN_POINT('Ctrl Pts',(73.3481561464184,-4.56469790617357,
78.2344304348218));
#181936=CARTESIAN_POINT('Ctrl Pts',(73.3938535732458,-4.59540760812734,
78.2276380224887));
#181937=CARTESIAN_POINT('Ctrl Pts',(73.6190821478091,-4.74186784983181,
78.1940037271525));
#181938=CARTESIAN_POINT('Ctrl Pts',(73.8046980317652,-4.84759864289241,
78.1658127326164));
#181939=CARTESIAN_POINT('Ctrl Pts',(74.2420269907349,-5.06360827697723,
78.0990593564817));
#181940=CARTESIAN_POINT('Ctrl Pts',(74.496801694948,-5.16618469854028,78.059950463295));
#181941=CARTESIAN_POINT('Ctrl Pts',(74.8445615408675,-5.27626147679226,
78.0068425413925));
#181942=CARTESIAN_POINT('Ctrl Pts',(74.9316261869138,-5.30142343629455,
77.9935659997728));
#181943=CARTESIAN_POINT('Ctrl Pts',(75.0886038253393,-5.34253034104682,
77.9696763487962));
#181944=CARTESIAN_POINT('Ctrl Pts',(75.1582824926091,-5.35929844186769,
77.9590888645066));
#181945=CARTESIAN_POINT('Ctrl Pts',(75.3134418479235,-5.39337657997133,
77.9355535623203));
#181946=CARTESIAN_POINT('Ctrl Pts',(75.3990488143221,-5.41001011726648,
77.9225954843572));
#181947=CARTESIAN_POINT('Ctrl Pts',(75.7102093890379,-5.46266031799454,
77.8755946931989));
#181948=CARTESIAN_POINT('Ctrl Pts',(75.9375781786611,-5.48639139088477,
77.8414483751284));
#181949=CARTESIAN_POINT('Ctrl Pts',(76.4717560240562,-5.50797522293383,
77.7614291770985));
#181950=CARTESIAN_POINT('Ctrl Pts',(76.7782687619571,-5.49420419072485,
77.7156823754374));
#181951=CARTESIAN_POINT('Ctrl Pts',(77.1390469762435,-5.44696380195649,
77.6612324020674));
#181952=CARTESIAN_POINT('Ctrl Pts',(77.196053242006,-5.43856610476701,77.6526094692588));
#181953=CARTESIAN_POINT('Ctrl Pts',(77.2908545206037,-5.4230409792205,77.6382272438688));
#181954=CARTESIAN_POINT('Ctrl Pts',(77.3287278389919,-5.41642103018427,
77.632469865077));
#181955=CARTESIAN_POINT('Ctrl Pts',(77.4138797709276,-5.40059452945907,
77.6194973246863));
#181956=CARTESIAN_POINT('Ctrl Pts',(77.4611114023374,-5.39115805624824,
77.6122831750434));
#181957=CARTESIAN_POINT('Ctrl Pts',(77.6281990785717,-5.3554358377391,77.5867110065965));
#181958=CARTESIAN_POINT('Ctrl Pts',(77.7472809501946,-5.32568489488279,
77.5683925200686));
#181959=CARTESIAN_POINT('Ctrl Pts',(78.1053770441845,-5.22310057412976,
77.5132174135964));
#181960=CARTESIAN_POINT('Ctrl Pts',(78.3405070859524,-5.13767354331611,
77.4768790226374));
#181961=CARTESIAN_POINT('Ctrl Pts',(78.7404301020967,-4.96013116249166,
77.415616902084));
#181962=CARTESIAN_POINT('Ctrl Pts',(78.9078309619874,-4.875156892705,77.3901504149331));
#181963=CARTESIAN_POINT('Ctrl Pts',(79.1453763270134,-4.73866867900507,
77.3544256550122));
#181964=CARTESIAN_POINT('Ctrl Pts',(79.2191314864121,-4.69392572879059,
77.3433938929701));
#181965=CARTESIAN_POINT('Ctrl Pts',(79.351830212482,-4.6090497848127,77.32366616379));
#181966=CARTESIAN_POINT('Ctrl Pts',(79.4111012832259,-4.5694813702983,77.3149001516919));
#181967=CARTESIAN_POINT('Ctrl Pts',(79.5450674680594,-4.47620387280451,
77.2951948048033));
#181968=CARTESIAN_POINT('Ctrl Pts',(79.6192254649066,-4.4217385150286,77.2843663292351));
#181969=CARTESIAN_POINT('Ctrl Pts',(79.8661236949224,-4.23062963903575,
77.2485833938717));
#181970=CARTESIAN_POINT('Ctrl Pts',(80.0321020875712,-4.0853500526018,77.2249996989916));
#181971=CARTESIAN_POINT('Ctrl Pts',(80.3770877452172,-3.74458755207061,
77.1768042557059));
#181972=CARTESIAN_POINT('Ctrl Pts',(80.5516846779828,-3.54530748027666,
77.1529849231373));
#181973=CARTESIAN_POINT('Ctrl Pts',(80.7449291807962,-3.289671324393,77.1268388796537));
#181974=CARTESIAN_POINT('Ctrl Pts',(80.7778337073023,-3.24474172580001,
77.1223948018454));
#181975=CARTESIAN_POINT('Ctrl Pts',(80.8342795116069,-3.16516024457205,
77.1147763120518));
#181976=CARTESIAN_POINT('Ctrl Pts',(80.8581152007823,-3.13072857974572,
77.1115601736501));
#181977=CARTESIAN_POINT('Ctrl Pts',(80.9159704515299,-3.04508198641242,
77.103757919598));
#181978=CARTESIAN_POINT('Ctrl Pts',(80.9495317145112,-2.99355997477047,
77.0992367451616));
#181979=CARTESIAN_POINT('Ctrl Pts',(81.0806542452679,-2.78471121802515,
77.0816257209535));
#181980=CARTESIAN_POINT('Ctrl Pts',(81.1711708943279,-2.62301976716516,
77.0695947879003));
#181981=CARTESIAN_POINT('Ctrl Pts',(81.3846939471021,-2.19232821640308,
77.0420862662766));
#181982=CARTESIAN_POINT('Ctrl Pts',(81.494668396106,-1.91739730959131,77.0288802362698));
#181983=CARTESIAN_POINT('Ctrl Pts',(81.6092575918458,-1.54846266234088,
77.0172939596629));
#181984=CARTESIAN_POINT('Ctrl Pts',(81.6340076070984,-1.46136286947176,
77.0149840412515));
#181985=CARTESIAN_POINT('Ctrl Pts',(81.6747303956036,-1.30358551011628,
77.0115720452801));
#181986=CARTESIAN_POINT('Ctrl Pts',(81.6914641784746,-1.23312949497981,
77.0103209662707));
#181987=CARTESIAN_POINT('Ctrl Pts',(81.7257212797353,-1.07534102745151,
77.0081278597913));
#181988=CARTESIAN_POINT('Ctrl Pts',(81.7425374873427,-0.987874062180328,
77.0073233186233));
#181989=CARTESIAN_POINT('Ctrl Pts',(81.7984979681635,-0.654057669637169,
77.0058079408019));
#181990=CARTESIAN_POINT('Ctrl Pts',(81.8232638414437,-0.405590901814358,
77.0078914150837));
#181991=CARTESIAN_POINT('Ctrl Pts',(81.8408767982921,0.136259595556882,
77.0190341318126));
#181992=CARTESIAN_POINT('Ctrl Pts',(81.8273896706965,0.429076623559226,
77.0292306958749));
#181993=CARTESIAN_POINT('Ctrl Pts',(81.7839324949371,0.775010049311216,
77.0455679559407));
#181994=CARTESIAN_POINT('Ctrl Pts',(81.7760903008232,0.830602387995591,
77.0483262831829));
#181995=CARTESIAN_POINT('Ctrl Pts',(81.7614262060612,0.924244870551358,
77.0531885307232));
#181996=CARTESIAN_POINT('Ctrl Pts',(81.7550476793131,0.962362850263627,
77.0552281602543));
#181997=CARTESIAN_POINT('Ctrl Pts',(81.7395031108337,1.04963382120321,77.0600357087681));
#181998=CARTESIAN_POINT('Ctrl Pts',(81.7300698954508,1.09873251147178,77.0628421610904));
#181999=CARTESIAN_POINT('Ctrl Pts',(81.6922889676162,1.28195922764356,77.0737136548726));
#182000=CARTESIAN_POINT('Ctrl Pts',(81.6596380006978,1.41510979657309,77.0824176659593));
#182001=CARTESIAN_POINT('Ctrl Pts',(81.5331782405383,1.85902405533254,77.1144528298743));
#182002=CARTESIAN_POINT('Ctrl Pts',(81.4171056511614,2.16245303430398,77.141466786713));
#182003=CARTESIAN_POINT('Ctrl Pts',(81.2172769762977,2.57296674037598,77.1865563833648));
#182004=CARTESIAN_POINT('Ctrl Pts',(81.1549207734837,2.69013927909417,77.2004816465146));
#182005=CARTESIAN_POINT('Ctrl Pts',(81.0496810078485,2.87178631257707,77.2238139688302));
#182006=CARTESIAN_POINT('Ctrl Pts',(81.0095262863717,2.93784854735424,77.2326820075019));
#182007=CARTESIAN_POINT('Ctrl Pts',(80.9280209391364,3.06578982023334,77.2506219619903));
#182008=CARTESIAN_POINT('Ctrl Pts',(80.8867771179038,3.12771983020459,77.2596724989083));
#182009=CARTESIAN_POINT('Ctrl Pts',(80.778955250213,3.28270065381025,77.2832663043536));
#182010=CARTESIAN_POINT('Ctrl Pts',(80.7107247356784,3.37450706614495,77.2981368225682));
#182011=CARTESIAN_POINT('Ctrl Pts',(80.5475752770769,3.58023758284994,77.333547134879));
#182012=CARTESIAN_POINT('Ctrl Pts',(80.4508235937867,3.69253015902679,77.3544434884665));
#182013=CARTESIAN_POINT('Ctrl Pts',(80.1524629299034,4.01151090457892,77.4184755616101));
#182014=CARTESIAN_POINT('Ctrl Pts',(79.9390498331029,4.20600000770045,77.4637937421474));
#182015=CARTESIAN_POINT('Ctrl Pts',(79.6688042917803,4.41523690861074,77.5199665530783));
#182016=CARTESIAN_POINT('Ctrl Pts',(79.6257502800877,4.44754849985687,77.528881276898));
#182017=CARTESIAN_POINT('Ctrl Pts',(79.5485442093124,4.50369564896925,77.5447984217472));
#182018=CARTESIAN_POINT('Ctrl Pts',(79.5145842482227,4.52779303181809,77.5517759230397));
#182019=CARTESIAN_POINT('Ctrl Pts',(79.4276978569702,4.58793715953203,77.569571052899));
#182020=CARTESIAN_POINT('Ctrl Pts',(79.3744066450802,4.62343102526966,77.5804341139877));
#182021=CARTESIAN_POINT('Ctrl Pts',(79.2511332780576,4.70238535303766,77.6054685321576));
#182022=CARTESIAN_POINT('Ctrl Pts',(79.1807663898367,4.74519842856199,77.6196914080793));
#182023=CARTESIAN_POINT('Ctrl Pts',(78.9103347465932,4.90130966127014,77.6741742056773));
#182024=CARTESIAN_POINT('Ctrl Pts',(78.7041753801489,5.00322003312319,77.7153569978125));
#182025=CARTESIAN_POINT('Ctrl Pts',(78.3327149916367,5.15793848190996,77.7895567050763));
#182026=CARTESIAN_POINT('Ctrl Pts',(78.1701091356487,5.21656711419243,77.8220339134506));
#182027=CARTESIAN_POINT('Ctrl Pts',(77.9256536568818,5.29149181960343,77.870983437678));
#182028=CARTESIAN_POINT('Ctrl Pts',(77.8457258618932,5.31395573612381,77.8870064885063));
#182029=CARTESIAN_POINT('Ctrl Pts',(77.6961658935369,5.35223292687144,77.9170324916188));
#182030=CARTESIAN_POINT('Ctrl Pts',(77.6266711965583,5.36853309543603,77.9310017037321));
#182031=CARTESIAN_POINT('Ctrl Pts',(77.4643084553455,5.40317598499173,77.9636822491622));
#182032=CARTESIAN_POINT('Ctrl Pts',(77.3712464870708,5.42044161914755,77.9824470464339));
#182033=CARTESIAN_POINT('Ctrl Pts',(77.0448123127249,5.47200266632727,78.0483814223472));
#182034=CARTESIAN_POINT('Ctrl Pts',(76.8097572798377,5.49318038295565,78.0960720442571));
#182035=CARTESIAN_POINT('Ctrl Pts',(76.2989801747345,5.50493167208876,78.199847677639));
#182036=CARTESIAN_POINT('Ctrl Pts',(76.0237871485224,5.48976380034184,78.2558521585353));
#182037=CARTESIAN_POINT('Ctrl Pts',(75.6956875849196,5.44584497720425,78.322100559458));
#182038=CARTESIAN_POINT('Ctrl Pts',(75.6406274761654,5.43758927256413,78.3331992247991));
#182039=CARTESIAN_POINT('Ctrl Pts',(75.5624980574765,5.42461269953035,78.3489132435704));
#182040=CARTESIAN_POINT('Ctrl Pts',(75.5393227029819,5.42060485865232,78.3535700775961));
#182041=CARTESIAN_POINT('Ctrl Pts',(75.5161728246847,5.41644264198492,78.358216968557));
#182042=CARTESIAN_POINT('Origin',(76.1212924379081,7.15881389286582E-15,
76.2900208433682));
#182043=CARTESIAN_POINT('',(75.1812918055742,5.62353578632127,76.6693002371056));
#182044=CARTESIAN_POINT('',(75.1807370437626,5.41644264156715,76.4558661362069));
#182045=CARTESIAN_POINT('',(75.1807370437626,5.41644264156718,76.4558661362069));
#182046=CARTESIAN_POINT('Ctrl Pts',(75.1812918055743,5.62353578632128,76.6693002371056));
#182047=CARTESIAN_POINT('Ctrl Pts',(75.3571628611358,5.65249493893739,76.6356794593437));
#182048=CARTESIAN_POINT('Ctrl Pts',(75.5392018334951,5.67354545131171,76.6007060003843));
#182049=CARTESIAN_POINT('Ctrl Pts',(76.4013260614393,5.72703701773099,76.4347216202953));
#182050=CARTESIAN_POINT('Ctrl Pts',(77.0795952398394,5.64345323809595,76.3037649317242));
#182051=CARTESIAN_POINT('Ctrl Pts',(78.3313431664491,5.25009364564398,76.0645802175305));
#182052=CARTESIAN_POINT('Ctrl Pts',(78.9730340238476,4.9347614241347,75.9433917035655));
#182053=CARTESIAN_POINT('Ctrl Pts',(80.1203906190512,3.99017560718347,75.7178789883305));
#182054=CARTESIAN_POINT('Ctrl Pts',(80.579679906946,3.43286338982664,75.6247561696959));
#182055=CARTESIAN_POINT('Ctrl Pts',(81.2545152194198,2.20195736568136,75.486134896178));
#182056=CARTESIAN_POINT('Ctrl Pts',(81.4757538887496,1.53878263947313,75.4394015224678));
#182057=CARTESIAN_POINT('Ctrl Pts',(81.6668477957519,0.11632693193044,75.3839335879276));
#182058=CARTESIAN_POINT('Ctrl Pts',(81.6175680342668,-0.63462652993374,
75.3793749075201));
#182059=CARTESIAN_POINT('Ctrl Pts',(81.301051587549,-1.82835714239946,75.4171500760812));
#182060=CARTESIAN_POINT('Ctrl Pts',(81.1132524101206,-2.28694413181046,
75.4439714552156));
#182061=CARTESIAN_POINT('Ctrl Pts',(80.5715823219023,-3.22898572750882,
75.5247634044448));
#182062=CARTESIAN_POINT('Ctrl Pts',(80.1950180370635,-3.68900287460553,
75.5813656397829));
#182063=CARTESIAN_POINT('Ctrl Pts',(79.7540569593757,-4.07954801327268,
75.6494664436731));
#182064=CARTESIAN_POINT('Origin',(76.1212924379081,7.15881389286582E-15,
76.2900208433682));
#182065=CARTESIAN_POINT('Origin',(76.5901425176087,7.15881389286582E-15,
78.9490017765011));
#182066=CARTESIAN_POINT('',(77.4871784401325,-5.90884651804035,78.0363452943797));
#182067=CARTESIAN_POINT('',(77.5021200054788,-5.908846518253,78.1210831292301));
#182068=CARTESIAN_POINT('',(77.6162029475856,-5.90884651807327,78.7680796388589));
#182069=CARTESIAN_POINT('',(79.5631824082914,5.13997981404828,77.9850820082636));
#182070=CARTESIAN_POINT('Ctrl Pts',(77.4871784403164,-5.90884651800743,
78.0363452943473));
#182071=CARTESIAN_POINT('Ctrl Pts',(77.4934521895834,-5.90772748441951,
78.0353782935762));
#182072=CARTESIAN_POINT('Ctrl Pts',(77.4997242490394,-5.90659822221011,
78.0344119531403));
#182073=CARTESIAN_POINT('Ctrl Pts',(77.5491905020832,-5.89760890063681,
78.0267937527027));
#182074=CARTESIAN_POINT('Ctrl Pts',(77.5923018430072,-5.88927441212067,
78.0201728980026));
#182075=CARTESIAN_POINT('Ctrl Pts',(77.7226204751505,-5.86256270962865,
78.0002086856151));
#182076=CARTESIAN_POINT('Ctrl Pts',(77.809521806952,-5.84268235841269,77.9869632148244));
#182077=CARTESIAN_POINT('Ctrl Pts',(78.0252391937274,-5.7881465162295,77.9542074513322));
#182078=CARTESIAN_POINT('Ctrl Pts',(78.1534159958275,-5.75106742878112,
77.9348553780247));
#182079=CARTESIAN_POINT('Ctrl Pts',(78.6427061846875,-5.59132845044584,
77.8612129409205));
#182080=CARTESIAN_POINT('Ctrl Pts',(78.9931348457252,-5.4379969721673,77.8088954667391));
#182081=CARTESIAN_POINT('Ctrl Pts',(79.4129114087173,-5.20356389190537,
77.7459651290228));
#182082=CARTESIAN_POINT('Ctrl Pts',(79.4980462611288,-5.15317808949757,
77.7331925421746));
#182083=CARTESIAN_POINT('Ctrl Pts',(79.6433710922886,-5.06217692221251,
77.7113713228665));
#182084=CARTESIAN_POINT('Ctrl Pts',(79.7041421115543,-5.02255065225972,
77.702240540578));
#182085=CARTESIAN_POINT('Ctrl Pts',(79.8313313603613,-4.93624736284486,
77.6831207384009));
#182086=CARTESIAN_POINT('Ctrl Pts',(79.897552498061,-4.88930027149069,77.6731601456358));
#182087=CARTESIAN_POINT('Ctrl Pts',(80.0901498220812,-4.74673485561338,
77.6441837217559));
#182088=CARTESIAN_POINT('Ctrl Pts',(80.2137244739563,-4.64737175146598,
77.6255808618117));
#182089=CARTESIAN_POINT('Ctrl Pts',(80.5288369694172,-4.37257703915636,
77.5782399702202));
#182090=CARTESIAN_POINT('Ctrl Pts',(80.7132224137751,-4.1892832444789,77.5506310886405));
#182091=CARTESIAN_POINT('Ctrl Pts',(80.9924998716715,-3.87301939500085,
77.5095547870779));
#182092=CARTESIAN_POINT('Ctrl Pts',(81.0948131596446,-3.7472518757893,77.4947003301369));
#182093=CARTESIAN_POINT('Ctrl Pts',(81.2246072081861,-3.57387616237588,
77.4762834899382));
#182094=CARTESIAN_POINT('Ctrl Pts',(81.2566377307307,-3.52986284709273,
77.4717767011675));
#182095=CARTESIAN_POINT('Ctrl Pts',(81.312165945205,-3.45135528198662,77.4640408238861));
#182096=CARTESIAN_POINT('Ctrl Pts',(81.3359062018732,-3.41704355013873,
77.4607601686717));
#182097=CARTESIAN_POINT('Ctrl Pts',(81.3930224251975,-3.33264237448964,
77.4529327861897));
#182098=CARTESIAN_POINT('Ctrl Pts',(81.4260131437731,-3.28229100154471,
77.4484673199118));
#182099=CARTESIAN_POINT('Ctrl Pts',(81.5725537188299,-3.05119213104776,
77.4288659407011));
#182100=CARTESIAN_POINT('Ctrl Pts',(81.677320234815,-2.86490582309567,77.4155082355322));
#182101=CARTESIAN_POINT('Ctrl Pts',(81.9134163786765,-2.38767722651736,
77.3866762038847));
#182102=CARTESIAN_POINT('Ctrl Pts',(82.0320958321311,-2.09106969004154,
77.3734149465394));
#182103=CARTESIAN_POINT('Ctrl Pts',(82.1547121581883,-1.69705771604075,
77.3611545792717));
#182104=CARTESIAN_POINT('Ctrl Pts',(82.1804442516329,-1.60708685192427,
77.3587043525596));
#182105=CARTESIAN_POINT('Ctrl Pts',(82.2224391880432,-1.44627382091367,
77.3549381448688));
#182106=CARTESIAN_POINT('Ctrl Pts',(82.2395289392392,-1.37567029102757,
77.3534914232994));
#182107=CARTESIAN_POINT('Ctrl Pts',(82.2736990591403,-1.22253129794907,
77.3507994870256));
#182108=CARTESIAN_POINT('Ctrl Pts',(82.2903364210679,-1.13991171112005,
77.3496238249134));
#182109=CARTESIAN_POINT('Ctrl Pts',(82.3361142348001,-0.885313129490639,
77.3468556273716));
#182110=CARTESIAN_POINT('Ctrl Pts',(82.3595718363196,-0.712397746788869,
77.3461610483572));
#182111=CARTESIAN_POINT('Ctrl Pts',(82.402715406588,-0.243874795976445,
77.3476055428851));
#182112=CARTESIAN_POINT('Ctrl Pts',(82.408293118046,0.0525237387862707,
77.3520427942016));
#182113=CARTESIAN_POINT('Ctrl Pts',(82.3838007757034,0.506370742700034,
77.3650091906455));
#182114=CARTESIAN_POINT('Ctrl Pts',(82.3690904705875,0.66425556221823,77.3706817941234));
#182115=CARTESIAN_POINT('Ctrl Pts',(82.3419435601632,0.86904777868197,77.3796994117668));
#182116=CARTESIAN_POINT('Ctrl Pts',(82.335056535245,0.91667522339289,77.3819147345167));
#182117=CARTESIAN_POINT('Ctrl Pts',(82.3216087622276,1.00250647421022,77.3861266843378));
#182118=CARTESIAN_POINT('Ctrl Pts',(82.3152452153003,1.04074023492962,77.3880822416725));
#182119=CARTESIAN_POINT('Ctrl Pts',(82.3002681380371,1.12572747446224,77.3926081813163));
#182120=CARTESIAN_POINT('Ctrl Pts',(82.2914721862968,1.17244325089226,77.3952164770578));
#182121=CARTESIAN_POINT('Ctrl Pts',(82.2603860777859,1.32755435044431,77.4042695384468));
#182122=CARTESIAN_POINT('Ctrl Pts',(82.2356979403902,1.4354175678313,77.4112059067286));
#182123=CARTESIAN_POINT('Ctrl Pts',(82.1607155729078,1.72629187302632,77.4315751118181));
#182124=CARTESIAN_POINT('Ctrl Pts',(82.1047858091582,1.9076439630321,77.4460891739514));
#182125=CARTESIAN_POINT('Ctrl Pts',(81.9400767786863,2.36427339477832,77.487011271427));
#182126=CARTESIAN_POINT('Ctrl Pts',(81.8194709552043,2.63455885330743,77.51545158445));
#182127=CARTESIAN_POINT('Ctrl Pts',(81.6320905608724,2.98289882791018,77.5575958409496));
#182128=CARTESIAN_POINT('Ctrl Pts',(81.5823899803663,3.06997711289707,77.5686253574343));
#182129=CARTESIAN_POINT('Ctrl Pts',(81.4928895464382,3.21801555221704,77.5882400410595));
#182130=CARTESIAN_POINT('Ctrl Pts',(81.4541110955956,3.27958791484473,77.596666319509));
#182131=CARTESIAN_POINT('Ctrl Pts',(81.3699763322677,3.40791459938609,77.6148025710048));
#182132=CARTESIAN_POINT('Ctrl Pts',(81.3243735934911,3.47448429263782,77.624550124217));
#182133=CARTESIAN_POINT('Ctrl Pts',(81.1874713180948,3.66587946582856,77.6535890136189));
#182134=CARTESIAN_POINT('Ctrl Pts',(81.0926848879001,3.78804420079668,77.6734188213446));
#182135=CARTESIAN_POINT('Ctrl Pts',(80.8487045941295,4.07839506728686,77.7239267062195));
#182136=CARTESIAN_POINT('Ctrl Pts',(80.694582061473,4.24198142973002,77.7553891078798));
#182137=CARTESIAN_POINT('Ctrl Pts',(80.3991994696675,4.52183268944643,77.8153456803641));
#182138=CARTESIAN_POINT('Ctrl Pts',(80.2610490253404,4.64108636151601,77.843271634565));
#182139=CARTESIAN_POINT('Ctrl Pts',(80.0684362233177,4.79238834770303,77.8822816653051));
#182140=CARTESIAN_POINT('Ctrl Pts',(80.0185312143735,4.83031934508719,77.8923956293884));
#182141=CARTESIAN_POINT('Ctrl Pts',(79.9351129166709,4.89164994381174,77.9093250132792));
#182142=CARTESIAN_POINT('Ctrl Pts',(79.9019340398087,4.91551591261988,77.9160648202313));
#182143=CARTESIAN_POINT('Ctrl Pts',(79.8362690312939,4.96172044490222,77.9294181415151));
#182144=CARTESIAN_POINT('Ctrl Pts',(79.8038015726767,4.98408157776601,77.9360267919065));
#182145=CARTESIAN_POINT('Ctrl Pts',(79.7027226245189,5.0522090204933,77.9566151012401));
#182146=CARTESIAN_POINT('Ctrl Pts',(79.6334017069684,5.09683847834765,77.9707543688887));
#182147=CARTESIAN_POINT('Ctrl Pts',(79.5631824082903,5.1399798140475,77.9850820082609));
#182148=CARTESIAN_POINT('',(81.9970266959657,2.23885090499482,77.5559295935053));
#182149=CARTESIAN_POINT('Origin',(76.5149506510185,7.15881389286582E-15,
78.5225675105249));
#182150=CARTESIAN_POINT('Ctrl Pts',(81.9970266959657,2.23885090499483,77.5559295935053));
#182151=CARTESIAN_POINT('Ctrl Pts',(82.1120050374136,1.94599933596432,77.5297243427407));
#182152=CARTESIAN_POINT('Ctrl Pts',(82.2040639554934,1.64432695163046,77.5077093270866));
#182153=CARTESIAN_POINT('Ctrl Pts',(82.2828902621182,1.28846521688186,77.4864579936355));
#182154=CARTESIAN_POINT('Ctrl Pts',(82.2929691014602,1.24017294726578,77.4836714598941));
#182155=CARTESIAN_POINT('Ctrl Pts',(82.3109829666165,1.14824548678766,77.4785448540955));
#182156=CARTESIAN_POINT('Ctrl Pts',(82.3190311682852,1.10463675326511,77.476188302615));
#182157=CARTESIAN_POINT('Ctrl Pts',(82.3333026734869,1.02223313768075,77.4718722996966));
#182158=CARTESIAN_POINT('Ctrl Pts',(82.3396289029045,0.983459828563357,
77.4698979720648));
#182159=CARTESIAN_POINT('Ctrl Pts',(82.3552794816357,0.881281097813429,
77.4648469028044));
#182160=CARTESIAN_POINT('Ctrl Pts',(82.3639753086168,0.81777966209688,77.4618613282563));
#182161=CARTESIAN_POINT('Ctrl Pts',(82.4037315616389,0.488678616768583,
77.4472143836427));
#182162=CARTESIAN_POINT('Ctrl Pts',(82.4182052778017,0.221261346282158,
77.4380997327589));
#182163=CARTESIAN_POINT('Ctrl Pts',(82.4126053820003,-0.254384290371704,
77.4274857011276));
#182164=CARTESIAN_POINT('Ctrl Pts',(82.3995023391387,-0.462231518467035,
77.4247481407553));
#182165=CARTESIAN_POINT('Ctrl Pts',(82.3592317702824,-0.813793276268081,
77.4235226438736));
#182166=CARTESIAN_POINT('Ctrl Pts',(82.3374726948974,-0.957933874065452,
77.4240054560567));
#182167=CARTESIAN_POINT('Ctrl Pts',(82.2957859411768,-1.17996338745491,
77.4263009428648));
#182168=CARTESIAN_POINT('Ctrl Pts',(82.2794390815815,-1.25847397791779,
77.4274173744936));
#182169=CARTESIAN_POINT('Ctrl Pts',(82.2451426538702,-1.40834202947021,
77.4301338396418));
#182170=CARTESIAN_POINT('Ctrl Pts',(82.2274398314377,-1.47974197471554,
77.4316860734008));
#182171=CARTESIAN_POINT('Ctrl Pts',(82.1859290517851,-1.63508876171119,
77.4356259025677));
#182172=CARTESIAN_POINT('Ctrl Pts',(82.16160312302,-1.71887716814351,77.4381148156318));
#182173=CARTESIAN_POINT('Ctrl Pts',(82.0314402667802,-2.13374512299529,
77.4522364787784));
#182174=CARTESIAN_POINT('Ctrl Pts',(81.8992835045091,-2.45568309340538,
77.4690056300341));
#182175=CARTESIAN_POINT('Ctrl Pts',(81.6540035372506,-2.93205429856277,
77.5019645828343));
#182176=CARTESIAN_POINT('Ctrl Pts',(81.5598497780608,-3.09561905023603,
77.514897877802));
#182177=CARTESIAN_POINT('Ctrl Pts',(81.4279559246922,-3.30170314609991,
77.5331169759468));
#182178=CARTESIAN_POINT('Ctrl Pts',(81.3970410614265,-3.34854956798892,
77.5373935803693));
#182179=CARTESIAN_POINT('Ctrl Pts',(81.3420287649319,-3.42942212812094,
77.5450050301176));
#182180=CARTESIAN_POINT('Ctrl Pts',(81.3182238189387,-3.46364501950419,
77.5482985021127));
#182181=CARTESIAN_POINT('Ctrl Pts',(81.259670078947,-3.5459803155784,77.5563995283866));
#182182=CARTESIAN_POINT('Ctrl Pts',(81.2245630794915,-3.59382662288795,
77.5612575885879));
#182183=CARTESIAN_POINT('Ctrl Pts',(81.0081907320452,-3.87972658424919,
77.5912365319937));
#182184=CARTESIAN_POINT('Ctrl Pts',(80.8101623365004,-4.10430694848959,
77.6188510676246));
#182185=CARTESIAN_POINT('Ctrl Pts',(80.4195031361362,-4.48573602355154,
77.6745915981231));
#182186=CARTESIAN_POINT('Ctrl Pts',(80.2321879254854,-4.64722355638303,
77.7017544178822));
#182187=CARTESIAN_POINT('Ctrl Pts',(79.9648059334976,-4.85026875973001,
77.7412735775394));
#182188=CARTESIAN_POINT('Ctrl Pts',(79.8928521612124,-4.90241442964863,
77.7519745563073));
#182189=CARTESIAN_POINT('Ctrl Pts',(79.7606804873029,-4.99376143995268,
77.7717508694137));
#182190=CARTESIAN_POINT('Ctrl Pts',(79.7008594761873,-5.03352412250738,
77.7807442290716));
#182191=CARTESIAN_POINT('Ctrl Pts',(79.5661937244769,-5.11955905971487,
77.8010814218768));
#182192=CARTESIAN_POINT('Ctrl Pts',(79.4910194599769,-5.16526692889563,
77.8124955658833));
#182193=CARTESIAN_POINT('Ctrl Pts',(79.2441170644402,-5.30796930960743,
77.8501674622348));
#182194=CARTESIAN_POINT('Ctrl Pts',(79.0686545369416,-5.3980175855351,77.8772243415634));
#182195=CARTESIAN_POINT('Ctrl Pts',(78.8710996987854,-5.48722382101834,
77.9078893790354));
#182196=CARTESIAN_POINT('Ctrl Pts',(78.8530349866649,-5.49527192125009,
77.910695184472));
#182197=CARTESIAN_POINT('Ctrl Pts',(78.5893178613139,-5.61117664038048,
77.9516791282966));
#182198=CARTESIAN_POINT('Ctrl Pts',(78.3368168404352,-5.7021663598798,77.9912323511788));
#182199=CARTESIAN_POINT('Ctrl Pts',(77.9530337472602,-5.81147711804384,
78.0511492520113));
#182200=CARTESIAN_POINT('Ctrl Pts',(77.8258375173985,-5.84314371042114,
78.0709726385734));
#182201=CARTESIAN_POINT('Ctrl Pts',(77.6490436772768,-5.88091734003757,
78.0983870894309));
#182202=CARTESIAN_POINT('Ctrl Pts',(77.6002634438982,-5.89069249364619,
78.1059367113938));
#182203=CARTESIAN_POINT('Ctrl Pts',(77.5349624918954,-5.90291613519415,
78.1160187700405));
#182204=CARTESIAN_POINT('Ctrl Pts',(77.5185474885862,-5.90591638755581,
78.1185510884974));
#182205=CARTESIAN_POINT('Ctrl Pts',(77.502120004475,-5.90884651843273,78.1210831294071));
#182206=CARTESIAN_POINT('Origin',(76.5901425176087,7.15881389286582E-15,
78.9490017765011));
#182207=CARTESIAN_POINT('',(77.348259898075,-5.90884651802685,77.24849909196));
#182208=CARTESIAN_POINT('',(77.3632014635974,-5.90884651820819,77.333236926787));
#182209=CARTESIAN_POINT('',(77.6162029475856,-5.90884651807327,78.7680796388589));
#182210=CARTESIAN_POINT('Ctrl Pts',(77.3482598983342,-5.90884651798042,
77.2484990919142));
#182211=CARTESIAN_POINT('Ctrl Pts',(77.3790711546296,-5.9033507881994,77.2437500164688));
#182212=CARTESIAN_POINT('Ctrl Pts',(77.4098401728518,-5.89760861672904,
77.2390170943833));
#182213=CARTESIAN_POINT('Ctrl Pts',(77.501562216025,-5.8797319940699,77.2249346127144));
#182214=CARTESIAN_POINT('Ctrl Pts',(77.562377308269,-5.86687515734464,77.2156321567381));
#182215=CARTESIAN_POINT('Ctrl Pts',(77.9405526013235,-5.78064123208494,
77.1579631435909));
#182216=CARTESIAN_POINT('Ctrl Pts',(78.2518151643068,-5.6819190906891,77.1112503853703));
#182217=CARTESIAN_POINT('Ctrl Pts',(78.7418618598244,-5.48044949971028,
77.0378262550683));
#182218=CARTESIAN_POINT('Ctrl Pts',(78.9261672244682,-5.39327789775599,
77.0102487576707));
#182219=CARTESIAN_POINT('Ctrl Pts',(79.2053686633304,-5.2430917088901,76.9684103040856));
#182220=CARTESIAN_POINT('Ctrl Pts',(79.3035235189632,-5.18660181413933,
76.9536905486092));
#182221=CARTESIAN_POINT('Ctrl Pts',(79.4635324694679,-5.08829686726246,
76.9296712579722));
#182222=CARTESIAN_POINT('Ctrl Pts',(79.5263106521541,-5.0480759154954,76.9202413710357));
#182223=CARTESIAN_POINT('Ctrl Pts',(79.6520127638248,-4.96415347527391,
76.9013491550527));
#182224=CARTESIAN_POINT('Ctrl Pts',(79.7148830134044,-4.92039526150578,
76.8918945994209));
#182225=CARTESIAN_POINT('Ctrl Pts',(79.879772149375,-4.80082632931245,76.8670902431858));
#182226=CARTESIAN_POINT('Ctrl Pts',(79.9802552595864,-4.72292066317286,
76.8519655210317));
#182227=CARTESIAN_POINT('Ctrl Pts',(80.3221192294778,-4.43986699813035,
76.8005508123697));
#182228=CARTESIAN_POINT('Ctrl Pts',(80.5497370329911,-4.21858474499515,
76.7663686369115));
#182229=CARTESIAN_POINT('Ctrl Pts',(80.8628864069086,-3.86167787207753,
76.7203560288381));
#182230=CARTESIAN_POINT('Ctrl Pts',(80.962123058527,-3.73917687711185,76.7059627377435));
#182231=CARTESIAN_POINT('Ctrl Pts',(81.0889456663203,-3.56943530517014,
76.6879779509928));
#182232=CARTESIAN_POINT('Ctrl Pts',(81.1208104650228,-3.52556740371241,
76.6834972089735));
#182233=CARTESIAN_POINT('Ctrl Pts',(81.1762065078811,-3.4471071564848,76.67578463301));
#182234=CARTESIAN_POINT('Ctrl Pts',(81.1999741205713,-3.41269244219758,
76.6725025375769));
#182235=CARTESIAN_POINT('Ctrl Pts',(81.2522757136796,-3.33525784369304,
76.6653401115408));
#182236=CARTESIAN_POINT('Ctrl Pts',(81.2806215533048,-3.29211181479248,
76.6614991886975));
#182237=CARTESIAN_POINT('Ctrl Pts',(81.4240819304952,-3.06754095051699,
76.6422570588391));
#182238=CARTESIAN_POINT('Ctrl Pts',(81.5301074658421,-2.88033546349416,
76.6287048894998));
#182239=CARTESIAN_POINT('Ctrl Pts',(81.7249388642508,-2.4891327612249,76.6048534090641));
#182240=CARTESIAN_POINT('Ctrl Pts',(81.8129408029566,-2.28508773182132,
76.5946877522053));
#182241=CARTESIAN_POINT('Ctrl Pts',(81.940405056024,-1.93830330023256,76.5808603903746));
#182242=CARTESIAN_POINT('Ctrl Pts',(81.9861923877244,-1.79816460303819,
76.5761677964281));
#182243=CARTESIAN_POINT('Ctrl Pts',(82.0489133782399,-1.57950915023936,
76.5701836645833));
#182244=CARTESIAN_POINT('Ctrl Pts',(82.0694669501074,-1.50210727408618,
76.5683186584049));
#182245=CARTESIAN_POINT('Ctrl Pts',(82.1059623572793,-1.3528193124491,76.5652046839765));
#182246=CARTESIAN_POINT('Ctrl Pts',(82.1221396477114,-1.28100642980992,
76.5639183685895));
#182247=CARTESIAN_POINT('Ctrl Pts',(82.1546220855387,-1.1235063695837,76.5615601922676));
#182248=CARTESIAN_POINT('Ctrl Pts',(82.1703950677187,-1.03772539479227,
76.560572045764));
#182249=CARTESIAN_POINT('Ctrl Pts',(82.2423549207679,-0.592700687420132,
76.5569926245351));
#182250=CARTESIAN_POINT('Ctrl Pts',(82.2680465566833,-0.229268870135951,
76.5591978923104));
#182251=CARTESIAN_POINT('Ctrl Pts',(82.2583380429672,0.286661204992796,
76.570595657831));
#182252=CARTESIAN_POINT('Ctrl Pts',(82.2497471197123,0.438962422474809,
76.5749939124982));
#182253=CARTESIAN_POINT('Ctrl Pts',(82.2263542662663,0.687645543165331,
76.5840166942483));
#182254=CARTESIAN_POINT('Ctrl Pts',(82.21492486286,0.784297601861131,76.5879833909021));
#182255=CARTESIAN_POINT('Ctrl Pts',(82.194768278483,0.925711463427947,76.5945026284016));
#182256=CARTESIAN_POINT('Ctrl Pts',(82.1878370007862,0.97073003571516,76.5966852322672));
#182257=CARTESIAN_POINT('Ctrl Pts',(82.1740671847905,1.05396961486788,76.6009251065495));
#182258=CARTESIAN_POINT('Ctrl Pts',(82.1673661448697,1.09221162697219,76.6029537339398));
#182259=CARTESIAN_POINT('Ctrl Pts',(82.1491895578466,1.19042655666336,76.6083690200036));
#182260=CARTESIAN_POINT('Ctrl Pts',(82.1371792745618,1.25029001896446,76.6118671338245));
#182261=CARTESIAN_POINT('Ctrl Pts',(82.064585414926,1.58590373360737,76.6325603162671));
#182262=CARTESIAN_POINT('Ctrl Pts',(81.9858403894899,1.85714328109069,76.6533951204252));
#182263=CARTESIAN_POINT('Ctrl Pts',(81.7910062878038,2.38682890637765,76.7015560127701));
#182264=CARTESIAN_POINT('Ctrl Pts',(81.6750623746765,2.64458181563327,76.7288350528002));
#182265=CARTESIAN_POINT('Ctrl Pts',(81.4939444286058,2.9815273686733,76.7695777129513));
#182266=CARTESIAN_POINT('Ctrl Pts',(81.444134851852,3.06884551453978,76.7806327997634));
#182267=CARTESIAN_POINT('Ctrl Pts',(81.3545084364918,3.21715114439041,76.8002767458305));
#182268=CARTESIAN_POINT('Ctrl Pts',(81.3157233773698,3.27875691452185,76.8087051014778));
#182269=CARTESIAN_POINT('Ctrl Pts',(81.2316536267014,3.40702916211221,76.826828574464));
#182270=CARTESIAN_POINT('Ctrl Pts',(81.1861272193596,3.4735142940962,76.8365605450676));
#182271=CARTESIAN_POINT('Ctrl Pts',(81.0498137022408,3.66417376553156,76.8654768613902));
#182272=CARTESIAN_POINT('Ctrl Pts',(80.9555866343288,3.78572443843611,76.8851924187907));
#182273=CARTESIAN_POINT('Ctrl Pts',(80.7003998580471,4.0898034979418,76.9380288313144));
#182274=CARTESIAN_POINT('Ctrl Pts',(80.5328346307177,4.26622038163841,76.9722003664408));
#182275=CARTESIAN_POINT('Ctrl Pts',(80.2298897979858,4.5482561867141,77.0336466448138));
#182276=CARTESIAN_POINT('Ctrl Pts',(80.0997635343139,4.65926376273859,77.0599520613209));
#182277=CARTESIAN_POINT('Ctrl Pts',(79.9179005993073,4.80125665779067,77.0967897013079));
#182278=CARTESIAN_POINT('Ctrl Pts',(79.8701275289562,4.83739855541433,77.1064731815232));
#182279=CARTESIAN_POINT('Ctrl Pts',(79.7885004244674,4.89721923095609,77.1230412699453));
#182280=CARTESIAN_POINT('Ctrl Pts',(79.7549253471949,4.92128628346686,77.1298628035971));
#182281=CARTESIAN_POINT('Ctrl Pts',(79.6763953948476,4.97633645073748,77.1458349046398));
#182282=CARTESIAN_POINT('Ctrl Pts',(79.6312636859136,5.00704651151342,77.1550258115393));
#182283=CARTESIAN_POINT('Ctrl Pts',(79.4443191832341,5.13047922390375,77.1931258300298));
#182284=CARTESIAN_POINT('Ctrl Pts',(79.2990614268771,5.21760201718711,77.2227964476991));
#182285=CARTESIAN_POINT('Ctrl Pts',(78.8117241196203,5.48183729584794,77.3221809444067));
#182286=CARTESIAN_POINT('Ctrl Pts',(78.4562563747846,5.63121342866614,77.3943578700479));
#182287=CARTESIAN_POINT('Ctrl Pts',(78.0064008746293,5.76960453436242,77.4844734985378));
#182288=CARTESIAN_POINT('Ctrl Pts',(77.9233625740266,5.79313209926972,77.501062917018));
#182289=CARTESIAN_POINT('Ctrl Pts',(77.777894583183,5.83085649495309,77.5300452579002));
#182290=CARTESIAN_POINT('Ctrl Pts',(77.7156930208904,5.84589101948722,77.5424131537475));
#182291=CARTESIAN_POINT('Ctrl Pts',(77.5702205906742,5.87850881592332,77.5712819966631));
#182292=CARTESIAN_POINT('Ctrl Pts',(77.4867883261293,5.89529187836198,77.5877963769558));
#182293=CARTESIAN_POINT('Ctrl Pts',(77.2150462302528,5.94374270511737,77.6414583094041));
#182294=CARTESIAN_POINT('Ctrl Pts',(77.0255479271987,5.96792495921637,77.678680261191));
#182295=CARTESIAN_POINT('Ctrl Pts',(76.445302374834,6.01293012420287,77.7923154695296));
#182296=CARTESIAN_POINT('Ctrl Pts',(76.053333974953,6.00353165605279,77.8685610020757));
#182297=CARTESIAN_POINT('Ctrl Pts',(75.5997939959963,5.9463772184808,77.9578966183986));
#182298=CARTESIAN_POINT('Ctrl Pts',(75.5343822295999,5.93699207884127,77.970810439319));
#182299=CARTESIAN_POINT('Ctrl Pts',(75.4339566251156,5.92082094221347,77.9906963290684));
#182300=CARTESIAN_POINT('Ctrl Pts',(75.3988199902583,5.91482902391477,77.9976652378463));
#182301=CARTESIAN_POINT('Ctrl Pts',(75.3232260793335,5.90121690882146,78.0126859086396));
#182302=CARTESIAN_POINT('Ctrl Pts',(75.2827902663125,5.89348866586959,78.0207376197063));
#182303=CARTESIAN_POINT('Ctrl Pts',(75.1689451325475,5.87046671645901,78.0434493967771));
#182304=CARTESIAN_POINT('Ctrl Pts',(75.0957444824899,5.85417517188175,78.05810281632));
#182305=CARTESIAN_POINT('Ctrl Pts',(74.9226081481883,5.81209155188762,78.0928541545413));
#182306=CARTESIAN_POINT('Ctrl Pts',(74.8229986862839,5.78503765703722,78.1129214145716));
#182307=CARTESIAN_POINT('Ctrl Pts',(74.5293644421938,5.69679239969982,78.1722195273797));
#182308=CARTESIAN_POINT('Ctrl Pts',(74.3377158148959,5.62800899289595,78.2111055782549));
#182309=CARTESIAN_POINT('Ctrl Pts',(73.9261607085401,5.45539875536574,78.2946849963179));
#182310=CARTESIAN_POINT('Ctrl Pts',(73.7082718840324,5.34754434783662,78.3389780652637));
#182311=CARTESIAN_POINT('Ctrl Pts',(73.4191050630308,5.1812115851068,78.3976619386656));
#182312=CARTESIAN_POINT('Ctrl Pts',(73.341734327806,5.13428885305903,78.4133549735778));
#182313=CARTESIAN_POINT('Ctrl Pts',(73.2051865571293,5.04709178188457,78.4410347683695));
#182314=CARTESIAN_POINT('Ctrl Pts',(73.1456133762532,5.00749883950254,78.4531053170519));
#182315=CARTESIAN_POINT('Ctrl Pts',(73.0174347482399,4.91889378656908,78.4790670253055));
#182316=CARTESIAN_POINT('Ctrl Pts',(72.9491218632164,4.86946900215564,78.4928971678718));
#182317=CARTESIAN_POINT('Ctrl Pts',(72.7314466994745,4.70474331056752,78.536960058539));
#182318=CARTESIAN_POINT('Ctrl Pts',(72.5864399036769,4.58365033245454,78.5662997403279));
#182319=CARTESIAN_POINT('Ctrl Pts',(72.2746137359892,4.29680075109632,78.6295654834212));
#182320=CARTESIAN_POINT('Ctrl Pts',(72.1112863269271,4.12758368576147,78.662824149951));
#182321=CARTESIAN_POINT('Ctrl Pts',(71.870254344542,3.84617123736604,78.7125617755189));
#182322=CARTESIAN_POINT('Ctrl Pts',(71.7857151199448,3.7403609422746,78.73015609352));
#182323=CARTESIAN_POINT('Ctrl Pts',(71.6739037977066,3.59016605858873,78.7537385413431));
#182324=CARTESIAN_POINT('Ctrl Pts',(71.6435215104869,3.54822145999234,78.7601811517279));
#182325=CARTESIAN_POINT('Ctrl Pts',(71.589675654306,3.47180237440665,78.7716704755811));
#182326=CARTESIAN_POINT('Ctrl Pts',(71.566021381508,3.43747108256943,78.776744092307));
#182327=CARTESIAN_POINT('Ctrl Pts',(71.5127759890861,3.35842654316031,78.7882281483384));
#182328=CARTESIAN_POINT('Ctrl Pts',(71.4834223271711,3.31355398678824,78.794604725575));
#182329=CARTESIAN_POINT('Ctrl Pts',(71.3731186550481,3.13986488387529,78.8187289731598));
#182330=CARTESIAN_POINT('Ctrl Pts',(71.2964613761757,3.00830213076517,78.8358416008123));
#182331=CARTESIAN_POINT('Ctrl Pts',(71.0699360511242,2.5830752296688,78.8873185155843));
#182332=CARTESIAN_POINT('Ctrl Pts',(70.9390316471772,2.27961473842733,78.9184716013972));
#182333=CARTESIAN_POINT('Ctrl Pts',(70.793741379226,1.84909333335007,78.9546378643439));
#182334=CARTESIAN_POINT('Ctrl Pts',(70.7576786172596,1.73032602313077,78.9638216683378));
#182335=CARTESIAN_POINT('Ctrl Pts',(70.7053089628792,1.53670177999723,78.9775127723781));
#182336=CARTESIAN_POINT('Ctrl Pts',(70.6867404453154,1.46252648723218,78.9824599568782));
#182337=CARTESIAN_POINT('Ctrl Pts',(70.6526329864705,1.31448581690629,78.9917455664844));
#182338=CARTESIAN_POINT('Ctrl Pts',(70.6370597010095,1.24064310023762,78.9960904558766));
#182339=CARTESIAN_POINT('Ctrl Pts',(70.6008859877896,1.05180481822983,79.0064782899364));
#182340=CARTESIAN_POINT('Ctrl Pts',(70.5822089173517,0.936453033749791,
79.0121459354762));
#182341=CARTESIAN_POINT('Ctrl Pts',(70.547647527451,0.675688201192122,79.0234691328582));
#182342=CARTESIAN_POINT('Ctrl Pts',(70.53365214637,0.530084714729527,79.0287602942883));
#182343=CARTESIAN_POINT('Ctrl Pts',(70.511168771355,0.1548468983974,79.0398650660739));
#182344=CARTESIAN_POINT('Ctrl Pts',(70.5103891421052,-0.0750483832367587,
79.0442424183622));
#182345=CARTESIAN_POINT('Ctrl Pts',(70.5316925031723,-0.474866480038174,
79.0480731938147));
#182346=CARTESIAN_POINT('Ctrl Pts',(70.5479368463135,-0.644820250329008,
79.0485043567766));
#182347=CARTESIAN_POINT('Ctrl Pts',(70.5787862245697,-0.867792083769855,
79.0476629821568));
#182348=CARTESIAN_POINT('Ctrl Pts',(70.5869736099093,-0.921619971103457,
79.0473508686733));
#182349=CARTESIAN_POINT('Ctrl Pts',(70.6021924541813,-1.01334267755272,
79.0466406735422));
#182350=CARTESIAN_POINT('Ctrl Pts',(70.6088619904773,-1.05129344331039,
79.0462947299494));
#182351=CARTESIAN_POINT('Ctrl Pts',(70.6249718461223,-1.13809376561228,
79.0453851293205));
#182352=CARTESIAN_POINT('Ctrl Pts',(70.6346524000807,-1.18689417817707,
79.0447866916639));
#182353=CARTESIAN_POINT('Ctrl Pts',(70.6712937973917,-1.3603896976341,79.0423369674326));
#182354=CARTESIAN_POINT('Ctrl Pts',(70.7015870666288,-1.48433981778062,
79.0399903856353));
#182355=CARTESIAN_POINT('Ctrl Pts',(70.8026000397794,-1.84762710450015,
79.0311950830383));
#182356=CARTESIAN_POINT('Ctrl Pts',(70.8841796742249,-2.08362081173422,
79.0229686366062));
#182357=CARTESIAN_POINT('Ctrl Pts',(71.0707862949551,-2.53207699382992,
79.0018369181684));
#182358=CARTESIAN_POINT('Ctrl Pts',(71.1742102788551,-2.74473498325315,
78.9892155731601));
#182359=CARTESIAN_POINT('Ctrl Pts',(71.3347443186164,-3.03105382907638,
78.968378600483));
#182360=CARTESIAN_POINT('Ctrl Pts',(71.3816118572124,-3.11035158702119,
78.9621745532778));
#182361=CARTESIAN_POINT('Ctrl Pts',(71.4684473269855,-3.2499071597528,78.9504723569842));
#182362=CARTESIAN_POINT('Ctrl Pts',(71.5077265158003,-3.31058312849762,
78.9451100350719));
#182363=CARTESIAN_POINT('Ctrl Pts',(71.5960936674664,-3.44186749178316,
78.932902427639));
#182364=CARTESIAN_POINT('Ctrl Pts',(71.6456162909299,-3.51215564211777,
78.9259704064296));
#182365=CARTESIAN_POINT('Ctrl Pts',(71.8146426493901,-3.74149126023436,
78.9020342531127));
#182366=CARTESIAN_POINT('Ctrl Pts',(71.9404454150299,-3.89559576849619,
78.8837807151736));
#182367=CARTESIAN_POINT('Ctrl Pts',(72.2297353203445,-4.21610106855887,
78.8411401613391));
#182368=CARTESIAN_POINT('Ctrl Pts',(72.3957240070386,-4.37973303814544,
78.816274006793));
#182369=CARTESIAN_POINT('Ctrl Pts',(72.6725242425283,-4.62236988992999,
78.7746531372064));
#182370=CARTESIAN_POINT('Ctrl Pts',(72.7772884530262,-4.70806953415733,
78.7588711913758));
#182371=CARTESIAN_POINT('Ctrl Pts',(72.9274027854656,-4.8225353462917,78.7363153631312));
#182372=CARTESIAN_POINT('Ctrl Pts',(72.9703847679667,-4.85440024466689,
78.7298634022445));
#182373=CARTESIAN_POINT('Ctrl Pts',(73.0475398544281,-4.9099972657163,78.7183013521376));
#182374=CARTESIAN_POINT('Ctrl Pts',(73.0815439835835,-4.93396034159707,
78.7132128792356));
#182375=CARTESIAN_POINT('Ctrl Pts',(73.1659269131394,-4.99210585650185,
78.7006021159989));
#182376=CARTESIAN_POINT('Ctrl Pts',(73.2165817224597,-5.02587092036607,
78.693045298111));
#182377=CARTESIAN_POINT('Ctrl Pts',(73.3311489404276,-5.09971428759275,
78.6759705361697));
#182378=CARTESIAN_POINT('Ctrl Pts',(73.3953215155522,-5.1393619065739,78.6664177369671));
#182379=CARTESIAN_POINT('Ctrl Pts',(73.6129231495262,-5.26812685262055,
78.6340284769649));
#182380=CARTESIAN_POINT('Ctrl Pts',(73.7695454363004,-5.35154195486914,
78.6107184103544));
#182381=CARTESIAN_POINT('Ctrl Pts',(74.1717066871822,-5.54305552232619,
78.5505973776636));
#182382=CARTESIAN_POINT('Ctrl Pts',(74.4212115348581,-5.64166994582414,
78.5130477600194));
#182383=CARTESIAN_POINT('Ctrl Pts',(74.7586908077126,-5.749142779127,78.4616710070052));
#182384=CARTESIAN_POINT('Ctrl Pts',(74.8415569552713,-5.77353818135924,
78.4490123123479));
#182385=CARTESIAN_POINT('Ctrl Pts',(74.9951687471143,-5.81511054217018,
78.4254640122467));
#182386=CARTESIAN_POINT('Ctrl Pts',(75.0657594516289,-5.83281585205253,
78.4146110837366));
#182387=CARTESIAN_POINT('Ctrl Pts',(75.2139053425179,-5.86706368554338,
78.3917698370917));
#182388=CARTESIAN_POINT('Ctrl Pts',(75.2915015900023,-5.88335551660229,
78.3797693840146));
#182389=CARTESIAN_POINT('Ctrl Pts',(75.5108846805038,-5.92479857874658,
78.3457453120744));
#182390=CARTESIAN_POINT('Ctrl Pts',(75.6532739912601,-5.94630716369097,
78.3235490851347));
#182391=CARTESIAN_POINT('Ctrl Pts',(76.0004674690265,-5.98574690419399,
78.2692264031445));
#182392=CARTESIAN_POINT('Ctrl Pts',(76.2056770401233,-5.99818481926721,
78.2369480187758));
#182393=CARTESIAN_POINT('Ctrl Pts',(76.6757119567096,-6.00191587115732,
78.1629755805831));
#182394=CARTESIAN_POINT('Ctrl Pts',(76.9401480940848,-5.98608198242611,
78.1213282851397));
#182395=CARTESIAN_POINT('Ctrl Pts',(77.2656229967027,-5.94435941151455,
78.0706370856789));
#182396=CARTESIAN_POINT('Ctrl Pts',(77.3283927806842,-5.93527647940671,
78.0608882287249));
#182397=CARTESIAN_POINT('Ctrl Pts',(77.4231095424685,-5.92000016877387,
78.046230927269));
#182398=CARTESIAN_POINT('Ctrl Pts',(77.4551659898521,-5.9145565019064,78.041279515172));
#182399=CARTESIAN_POINT('Ctrl Pts',(77.4871784403164,-5.90884651800743,
78.0363452943473));
#182400=CARTESIAN_POINT('Ctrl Pts',(77.502120004475,-5.90884651843273,78.1210831294071));
#182401=CARTESIAN_POINT('Ctrl Pts',(77.4810781240556,-5.91259970809392,
78.1243264076644));
#182402=CARTESIAN_POINT('Ctrl Pts',(77.4600157665999,-5.91623785047641,
78.1275692307462));
#182403=CARTESIAN_POINT('Ctrl Pts',(77.38652458514,-5.92851876326947,78.138872518064));
#182404=CARTESIAN_POINT('Ctrl Pts',(77.3339985198352,-5.9365641204623,78.1469306821317));
#182405=CARTESIAN_POINT('Ctrl Pts',(77.1211780008003,-5.96620813885608,
78.1795132683561));
#182406=CARTESIAN_POINT('Ctrl Pts',(76.9601266461478,-5.981887537296,78.2040189643669));
#182407=CARTESIAN_POINT('Ctrl Pts',(76.5105549554249,-6.00696129925713,
78.2722875244955));
#182408=CARTESIAN_POINT('Ctrl Pts',(76.2216665999468,-6.0017606095316,78.3160155976274));
#182409=CARTESIAN_POINT('Ctrl Pts',(75.7637031404583,-5.95963661516321,
78.3856978496139));
#182410=CARTESIAN_POINT('Ctrl Pts',(75.5938297520057,-5.93647412939509,
78.4116204353954));
#182411=CARTESIAN_POINT('Ctrl Pts',(75.3433402575683,-5.8910709563988,78.4499957144422));
#182412=CARTESIAN_POINT('Ctrl Pts',(75.2618009254828,-5.87449363876011,
78.4625111231067));
#182413=CARTESIAN_POINT('Ctrl Pts',(75.1105319573522,-5.84037625291913,
78.4857723924628));
#182414=CARTESIAN_POINT('Ctrl Pts',(75.0407197676059,-5.82327804644709,
78.4965250099047));
#182415=CARTESIAN_POINT('Ctrl Pts',(74.8815225455768,-5.78117587108564,
78.5210809497447));
#182416=CARTESIAN_POINT('Ctrl Pts',(74.7923774225082,-5.75532525174935,
78.5348579223328));
#182417=CARTESIAN_POINT('Ctrl Pts',(74.4060712149261,-5.63331180874198,
78.5946473582739));
#182418=CARTESIAN_POINT('Ctrl Pts',(74.1161143044717,-5.51562633175389,
78.6397838540036));
#182419=CARTESIAN_POINT('Ctrl Pts',(73.6468058642806,-5.28019114583707,
78.7124137024077));
#182420=CARTESIAN_POINT('Ctrl Pts',(73.4621587323749,-5.17475206926377,
78.7408586373746));
#182421=CARTESIAN_POINT('Ctrl Pts',(73.2321074079956,-5.0264736214097,78.775795459682));
#182422=CARTESIAN_POINT('Ctrl Pts',(73.1812939893964,-4.99260329560031,
78.7834786146529));
#182423=CARTESIAN_POINT('Ctrl Pts',(73.0967382406848,-4.93434360302729,
78.7961950097605));
#182424=CARTESIAN_POINT('Ctrl Pts',(73.0627215504062,-4.91037663159999,
78.8012912367867));
#182425=CARTESIAN_POINT('Ctrl Pts',(72.9856581580757,-4.85486450461443,
78.8127897631209));
#182426=CARTESIAN_POINT('Ctrl Pts',(72.9427758341716,-4.82309218052059,
78.8191552554317));
#182427=CARTESIAN_POINT('Ctrl Pts',(72.7931050519905,-4.7090566090581,78.8412692764551));
#182428=CARTESIAN_POINT('Ctrl Pts',(72.6886349444853,-4.62372059008446,
78.8565169546274));
#182429=CARTESIAN_POINT('Ctrl Pts',(72.4039859753521,-4.37467338128644,
78.8976814089308));
#182430=CARTESIAN_POINT('Ctrl Pts',(72.2306731758408,-4.20330302562194,
78.9222989569011));
#182431=CARTESIAN_POINT('Ctrl Pts',(71.9405115839662,-3.87909173876399,
78.9630949173958));
#182432=CARTESIAN_POINT('Ctrl Pts',(71.8196909512825,-3.73034426439076,
78.9799252905244));
#182433=CARTESIAN_POINT('Ctrl Pts',(71.6556021569751,-3.50731890321708,
79.0026172808806));
#182434=CARTESIAN_POINT('Ctrl Pts',(71.6065277460403,-3.43755535910792,
79.0093788895633));
#182435=CARTESIAN_POINT('Ctrl Pts',(71.5186060903433,-3.30673921365021,
79.0214467493572));
#182436=CARTESIAN_POINT('Ctrl Pts',(71.4793467394119,-3.24598871286321,
79.0268167850708));
#182437=CARTESIAN_POINT('Ctrl Pts',(71.3929507637437,-3.10686101821857,
79.0385889666235));
#182438=CARTESIAN_POINT('Ctrl Pts',(71.3464815763088,-3.02808218467929,
79.0448879448201));
#182439=CARTESIAN_POINT('Ctrl Pts',(71.1732662685583,-2.71854836124091,
79.0682170633539));
#182440=CARTESIAN_POINT('Ctrl Pts',(71.059826609919,-2.48053914474249,79.0831758788176));
#182441=CARTESIAN_POINT('Ctrl Pts',(70.87762297681,-2.02378725445234,79.1060554196966));
#182442=CARTESIAN_POINT('Ctrl Pts',(70.8050609226306,-1.8071080843895,79.1146268697831));
#182443=CARTESIAN_POINT('Ctrl Pts',(70.7125899545345,-1.46899309363459,
79.1241600181274));
#182444=CARTESIAN_POINT('Ctrl Pts',(70.6839124547786,-1.35022793137998,
79.1268028904188));
#182445=CARTESIAN_POINT('Ctrl Pts',(70.6487186515115,-1.18262561859743,
79.1294800780258));
#182446=CARTESIAN_POINT('Ctrl Pts',(70.6392080797634,-1.13445836139378,
79.1301289722111));
#182447=CARTESIAN_POINT('Ctrl Pts',(70.6232574819972,-1.04823304989988,
79.131069623875));
#182448=CARTESIAN_POINT('Ctrl Pts',(70.6165963389618,-1.01022021113656,
79.1314075839071));
#182449=CARTESIAN_POINT('Ctrl Pts',(70.6012615705156,-0.917569688070223,
79.1320459311201));
#182450=CARTESIAN_POINT('Ctrl Pts',(70.5929680129487,-0.862872580580845,
79.1322671359214));
#182451=CARTESIAN_POINT('Ctrl Pts',(70.5627346772902,-0.643450582698795,
79.1325498134125));
#182452=CARTESIAN_POINT('Ctrl Pts',(70.5467657719953,-0.477974560331505,
79.1314044998789));
#182453=CARTESIAN_POINT('Ctrl Pts',(70.521663444057,-0.0251427074124011,
79.1248599627512));
#182454=CARTESIAN_POINT('Ctrl Pts',(70.5260487930265,0.262494154087383,
79.1169911629691));
#182455=CARTESIAN_POINT('Ctrl Pts',(70.5655475721158,0.719976509478051,
79.0990956027503));
#182456=CARTESIAN_POINT('Ctrl Pts',(70.5876117910516,0.890583935872148,
79.0912035618539));
#182457=CARTESIAN_POINT('Ctrl Pts',(70.6311727026352,1.14260324412469,79.0777610855297));
#182458=CARTESIAN_POINT('Ctrl Pts',(70.6471684543172,1.22492153072512,79.0730821924442));
#182459=CARTESIAN_POINT('Ctrl Pts',(70.6801838701324,1.37779463145153,79.0638525873169));
#182460=CARTESIAN_POINT('Ctrl Pts',(70.6967740834076,1.44843046558834,79.0593699300092));
#182461=CARTESIAN_POINT('Ctrl Pts',(70.7377323678504,1.60972366911964,79.0486279769844));
#182462=CARTESIAN_POINT('Ctrl Pts',(70.7629472190068,1.70013719355725,79.0422355131372));
#182463=CARTESIAN_POINT('Ctrl Pts',(70.8805364802515,2.08674377854459,79.0132655185377));
#182464=CARTESIAN_POINT('Ctrl Pts',(70.9934843634689,2.37592268581678,78.9874405353129));
#182465=CARTESIAN_POINT('Ctrl Pts',(71.2229170769758,2.85166682606951,78.9368555082872));
#182466=CARTESIAN_POINT('Ctrl Pts',(71.3284077329428,3.04302851677477,78.9140470136933));
#182467=CARTESIAN_POINT('Ctrl Pts',(71.4760285704928,3.27944355035933,78.8822923739797));
#182468=CARTESIAN_POINT('Ctrl Pts',(71.5088874030224,3.33033713097156,78.8752327065569));
#182469=CARTESIAN_POINT('Ctrl Pts',(71.5655851247415,3.41530682124252,78.8630539710332));
#182470=CARTESIAN_POINT('Ctrl Pts',(71.5890239088569,3.44965503660483,78.858019595707));
#182471=CARTESIAN_POINT('Ctrl Pts',(71.6435649328426,3.5278250279607,78.8463038884903));
#182472=CARTESIAN_POINT('Ctrl Pts',(71.6748987077456,3.57147175199422,78.8395735696086));
#182473=CARTESIAN_POINT('Ctrl Pts',(71.7875306116366,3.72398881884504,78.815396461354));
#182474=CARTESIAN_POINT('Ctrl Pts',(71.8718967596723,3.83044081293952,78.7973152906231));
#182475=CARTESIAN_POINT('Ctrl Pts',(72.1173743245025,4.1193241886586,78.7449465808484));
#182476=CARTESIAN_POINT('Ctrl Pts',(72.2860272109715,4.2947358349363,78.7092428954034));
#182477=CARTESIAN_POINT('Ctrl Pts',(72.6029311674239,4.58606108534071,78.6430380342528));
#182478=CARTESIAN_POINT('Ctrl Pts',(72.746917174894,4.70626857602331,78.6132358570681));
#182479=CARTESIAN_POINT('Ctrl Pts',(72.9634341270755,4.87011521940609,78.5688789991628));
#182480=CARTESIAN_POINT('Ctrl Pts',(73.0316353584405,4.91945385069203,78.5549676410381));
#182481=CARTESIAN_POINT('Ctrl Pts',(73.1597199523187,5.00797520060226,78.5289533627614));
#182482=CARTESIAN_POINT('Ctrl Pts',(73.2193106901141,5.04756568761081,78.5168933569081));
#182483=CARTESIAN_POINT('Ctrl Pts',(73.3560480084358,5.13483989891192,78.4893145598342));
#182484=CARTESIAN_POINT('Ctrl Pts',(73.4335998210645,5.18183611589787,78.473739092791));
#182485=CARTESIAN_POINT('Ctrl Pts',(73.8472898215732,5.41954965747258,78.3909712517236));
#182486=CARTESIAN_POINT('Ctrl Pts',(74.2002983826242,5.57814411593327,78.3215025719002));
#182487=CARTESIAN_POINT('Ctrl Pts',(74.6972246977593,5.74441791578092,78.2238544198736));
#182488=CARTESIAN_POINT('Ctrl Pts',(74.8299523029251,5.7836151406408,78.1977768096684));
#182489=CARTESIAN_POINT('Ctrl Pts',(75.0520380985231,5.84065928275357,78.1540273375639));
#182490=CARTESIAN_POINT('Ctrl Pts',(75.1406763966927,5.86121586993014,78.1365360630712));
#182491=CARTESIAN_POINT('Ctrl Pts',(75.2728302167312,5.88860389802947,78.1103785416352));
#182492=CARTESIAN_POINT('Ctrl Pts',(75.3160189773529,5.8970424523266,78.1018176240498));
#182493=CARTESIAN_POINT('Ctrl Pts',(75.3970911722438,5.91192600531271,78.0857189003032));
#182494=CARTESIAN_POINT('Ctrl Pts',(75.4349516088338,5.91848767271836,78.0781888264813));
#182495=CARTESIAN_POINT('Ctrl Pts',(75.5339014319438,5.934623700944,78.058480720372));
#182496=CARTESIAN_POINT('Ctrl Pts',(75.5950776266932,5.94359557818371,78.0462686714658));
#182497=CARTESIAN_POINT('Ctrl Pts',(75.9757280691111,5.99319809033613,77.9701531281212));
#182498=CARTESIAN_POINT('Ctrl Pts',(76.2977978117972,6.00802499345337,77.9052178004773));
#182499=CARTESIAN_POINT('Ctrl Pts',(76.8195846727865,5.98838131167724,77.8002835312188));
#182500=CARTESIAN_POINT('Ctrl Pts',(77.0192096687312,5.97043414084938,77.7601943237206));
#182501=CARTESIAN_POINT('Ctrl Pts',(77.3294097530175,5.92619233449805,77.6981085906362));
#182502=CARTESIAN_POINT('Ctrl Pts',(77.4407802797377,5.90696307478835,77.6758595635005));
#182503=CARTESIAN_POINT('Ctrl Pts',(77.6239732150371,5.8697771405178,77.6393361917661));
#182504=CARTESIAN_POINT('Ctrl Pts',(77.6961242916996,5.85368736183456,77.6249704165238));
#182505=CARTESIAN_POINT('Ctrl Pts',(77.8413934735073,5.81836088217616,77.5960830339961));
#182506=CARTESIAN_POINT('Ctrl Pts',(77.9144839370153,5.79906566072541,77.5815677452047));
#182507=CARTESIAN_POINT('Ctrl Pts',(78.1068734326261,5.74423246994479,77.5434041952723));
#182508=CARTESIAN_POINT('Ctrl Pts',(78.2254723420467,5.70626788348198,77.519923810019));
#182509=CARTESIAN_POINT('Ctrl Pts',(78.6574950837772,5.5525025884081,77.4344842268919));
#182510=CARTESIAN_POINT('Ctrl Pts',(78.9623111365041,5.41346751704915,77.3744216644624));
#182511=CARTESIAN_POINT('Ctrl Pts',(79.3764899869024,5.17966590290425,77.2920348161791));
#182512=CARTESIAN_POINT('Ctrl Pts',(79.4966476933306,5.10599116173046,77.2680262770202));
#182513=CARTESIAN_POINT('Ctrl Pts',(79.6576903960397,4.99905313457317,77.2355871212688));
#182514=CARTESIAN_POINT('Ctrl Pts',(79.7009208729756,4.96950313728936,77.226852099324));
#182515=CARTESIAN_POINT('Ctrl Pts',(79.777747666932,4.91546146768861,77.2112717208417));
#182516=CARTESIAN_POINT('Ctrl Pts',(79.8114875006111,4.89118692514048,77.2044084912291));
#182517=CARTESIAN_POINT('Ctrl Pts',(79.895823206784,4.82913759845088,77.1872024718257));
#182518=CARTESIAN_POINT('Ctrl Pts',(79.9460778900933,4.7908962215886,77.1769035287751));
#182519=CARTESIAN_POINT('Ctrl Pts',(80.1635838218191,4.61977149189244,77.1321536635723));
#182520=CARTESIAN_POINT('Ctrl Pts',(80.324250531467,4.47853374837999,77.0986403117906));
#182521=CARTESIAN_POINT('Ctrl Pts',(80.6271125494264,4.18164522231204,77.0349406725622));
#182522=CARTESIAN_POINT('Ctrl Pts',(80.7693767387962,4.02650400762146,77.0047506848111));
#182523=CARTESIAN_POINT('Ctrl Pts',(80.9464266728784,3.81158112524013,76.9669685334703));
#182524=CARTESIAN_POINT('Ctrl Pts',(80.988708242165,3.75843012390612,76.9579275000913));
#182525=CARTESIAN_POINT('Ctrl Pts',(81.094494076567,3.62068772935883,76.935265544543));
#182526=CARTESIAN_POINT('Ctrl Pts',(81.1566958367114,3.53508461845458,76.9219001376667));
#182527=CARTESIAN_POINT('Ctrl Pts',(81.2581845445671,3.38733004669684,76.9000287062213));
#182528=CARTESIAN_POINT('Ctrl Pts',(81.2986414263839,3.32604764074379,76.8912909143801));
#182529=CARTESIAN_POINT('Ctrl Pts',(81.3801382552093,3.19752908873205,76.873647889353));
#182530=CARTESIAN_POINT('Ctrl Pts',(81.4210032529613,3.13019425222693,76.8647774825469));
#182531=CARTESIAN_POINT('Ctrl Pts',(81.5302614429409,2.94192024819869,76.8409875721766));
#182532=CARTESIAN_POINT('Ctrl Pts',(81.595837516978,2.81933548504786,76.8266243436442));
#182533=CARTESIAN_POINT('Ctrl Pts',(81.8163083064221,2.37053073248376,76.7779182144174));
#182534=CARTESIAN_POINT('Ctrl Pts',(81.9462949306246,2.0324542334475,76.7484150510847));
#182535=CARTESIAN_POINT('Ctrl Pts',(82.0860301786864,1.54156316515938,76.7140107508896));
#182536=CARTESIAN_POINT('Ctrl Pts',(82.1214375435231,1.39718988972072,76.7048636066006));
#182537=CARTESIAN_POINT('Ctrl Pts',(82.1619880194072,1.20078932387463,76.6935951612618));
#182538=CARTESIAN_POINT('Ctrl Pts',(82.1718276334386,1.14982724721509,76.6907763887375));
#182539=CARTESIAN_POINT('Ctrl Pts',(82.1878037718395,1.06094329259262,76.6860353501978));
#182540=CARTESIAN_POINT('Ctrl Pts',(82.1942371025926,1.02308124160296,76.6840703902107));
#182541=CARTESIAN_POINT('Ctrl Pts',(82.2083632519552,0.934859770359395,
76.6796183635456));
#182542=CARTESIAN_POINT('Ctrl Pts',(82.2157814810488,0.884458353110544,
76.6771710938632));
#182543=CARTESIAN_POINT('Ctrl Pts',(82.2402686356171,0.702136256874164,
76.6686771064589));
#182544=CARTESIAN_POINT('Ctrl Pts',(82.253628329319,0.569729862771318,76.6631852551421));
#182545=CARTESIAN_POINT('Ctrl Pts',(82.2784185771159,0.20409861249248,76.6500244617369));
#182546=CARTESIAN_POINT('Ctrl Pts',(82.2807799093679,-0.0295626711262976,
76.6438537772989));
#182547=CARTESIAN_POINT('Ctrl Pts',(82.2618435769026,-0.429656464211375,
76.6374850989974));
#182548=CARTESIAN_POINT('Ctrl Pts',(82.2471003818093,-0.596109657678972,
76.6360872992544));
#182549=CARTESIAN_POINT('Ctrl Pts',(82.2091099180954,-0.888187784942348,
76.6359207005032));
#182550=CARTESIAN_POINT('Ctrl Pts',(82.1887110791273,-1.01407673316437,
76.6366073461182));
#182551=CARTESIAN_POINT('Ctrl Pts',(82.1496475626092,-1.21509340448372,
76.6389362792751));
#182552=CARTESIAN_POINT('Ctrl Pts',(82.133467177538,-1.29066879784691,76.6400952949064));
#182553=CARTESIAN_POINT('Ctrl Pts',(82.0989573437285,-1.43812881980057,
76.642912701163));
#182554=CARTESIAN_POINT('Ctrl Pts',(82.0807435178298,-1.51002677651945,
76.6445488752448));
#182555=CARTESIAN_POINT('Ctrl Pts',(82.0313831230445,-1.69095525957267,
76.6493277639895));
#182556=CARTESIAN_POINT('Ctrl Pts',(81.9985020893052,-1.79947293740234,
76.6528089312253));
#182557=CARTESIAN_POINT('Ctrl Pts',(81.9175082166549,-2.04216298327549,
76.6619633365268));
#182558=CARTESIAN_POINT('Ctrl Pts',(81.8676790502401,-2.17567721545636,
76.6679676089574));
#182559=CARTESIAN_POINT('Ctrl Pts',(81.679944505087,-2.62934070051116,76.6916039852982));
#182560=CARTESIAN_POINT('Ctrl Pts',(81.5193074149887,-2.93907591727265,
76.7134752678841));
#182561=CARTESIAN_POINT('Ctrl Pts',(81.300880019114,-3.28356934743988,76.743633219079));
#182562=CARTESIAN_POINT('Ctrl Pts',(81.26804731515,-3.33367980522927,76.7481743819701));
#182563=CARTESIAN_POINT('Ctrl Pts',(81.2110942589947,-3.41782967137207,
76.7560540634447));
#182564=CARTESIAN_POINT('Ctrl Pts',(81.1873569589511,-3.45212657124492,
76.7593384248907));
#182565=CARTESIAN_POINT('Ctrl Pts',(81.1311145705204,-3.53160460917959,
76.7671194910825));
#182566=CARTESIAN_POINT('Ctrl Pts',(81.0983370790566,-3.57658288754655,
76.7716546612521));
#182567=CARTESIAN_POINT('Ctrl Pts',(80.9572400205273,-3.76464870121624,
76.7911976352345));
#182568=CARTESIAN_POINT('Ctrl Pts',(80.8431966105938,-3.90323958614348,
76.807045383938));
#182569=CARTESIAN_POINT('Ctrl Pts',(80.4697695933691,-4.31770968784781,
76.8594890092059));
#182570=CARTESIAN_POINT('Ctrl Pts',(80.1905711106454,-4.5740449840216,76.8995081864004));
#182571=CARTESIAN_POINT('Ctrl Pts',(79.819426840938,-4.85499887651365,76.9543868997662));
#182572=CARTESIAN_POINT('Ctrl Pts',(79.7482501543278,-4.9064451016579,76.9649759886891));
#182573=CARTESIAN_POINT('Ctrl Pts',(79.6168402424332,-4.99707237235025,
76.9846435149406));
#182574=CARTESIAN_POINT('Ctrl Pts',(79.5569772963478,-5.03677689086184,
76.9936454847934));
#182575=CARTESIAN_POINT('Ctrl Pts',(79.4213475048184,-5.1232370496266,77.0141332886399));
#182576=CARTESIAN_POINT('Ctrl Pts',(79.3452276705649,-5.16938833648931,
77.0256944149413));
#182577=CARTESIAN_POINT('Ctrl Pts',(79.0730678742054,-5.32613513134418,
77.067233631847));
#182578=CARTESIAN_POINT('Ctrl Pts',(78.8719291333387,-5.4271895740849,77.098305064101));
#182579=CARTESIAN_POINT('Ctrl Pts',(78.4557044736368,-5.60734040904606,
77.1630302216307));
#182580=CARTESIAN_POINT('Ctrl Pts',(78.2407864104021,-5.68586241316359,
77.1966643107356));
#182581=CARTESIAN_POINT('Ctrl Pts',(77.8754000295744,-5.795686413567,77.2537453323072));
#182582=CARTESIAN_POINT('Ctrl Pts',(77.727247794333,-5.83397582908958,77.2768607482368));
#182583=CARTESIAN_POINT('Ctrl Pts',(77.5314975681942,-5.8764784791733,77.3072295801729));
#182584=CARTESIAN_POINT('Ctrl Pts',(77.4850966509068,-5.88596643852881,
77.3144155863192));
#182585=CARTESIAN_POINT('Ctrl Pts',(77.4134884056225,-5.89970727127574,
77.3254808150766));
#182586=CARTESIAN_POINT('Ctrl Pts',(77.3883598281107,-5.90435908116652,
77.3293591566146));
#182587=CARTESIAN_POINT('Ctrl Pts',(77.3632014628439,-5.90884651834311,
77.3332369269199));
#182588=CARTESIAN_POINT('Origin',(79.767904168913,7.105427357601E-15,96.9709836566246));
#182589=CARTESIAN_POINT('',(78.0997797390488,-6.8936542710855,80.5105799046739));
#182590=CARTESIAN_POINT('Origin',(76.9027092374091,7.105427357601E-15,80.7216557319231));
#182591=CARTESIAN_POINT('',(80.8781505817192,-6.89365427108549,96.2675039528693));
#182592=CARTESIAN_POINT('',(80.9649746705526,-6.89365427108549,96.7599078293754));
#182593=CARTESIAN_POINT('',(74.7871667585286,-4.93000669486554,97.3415087399564));
#182594=CARTESIAN_POINT('Origin',(79.6810800800795,7.105427357601E-15,96.4785797801185));
#182595=CARTESIAN_POINT('',(74.3530463143613,-4.93000669486554,94.8794893574259));
#182596=CARTESIAN_POINT('',(74.873990847362,-4.93000669486554,97.8339126164625));
#182597=CARTESIAN_POINT('',(72.9876403879442,2.93305265169617,95.1202472618724));
#182598=CARTESIAN_POINT('Origin',(79.2469596359123,7.105427357601E-15,94.016560397588));
#182599=CARTESIAN_POINT('',(73.4217608321114,2.93305265169629,97.5822666444029));
#182600=CARTESIAN_POINT('',(73.5085849209449,2.93305265169617,98.074670520909));
#182601=CARTESIAN_POINT('',(84.5749934016305,4.93000669486556,95.6156508202806));
#182602=CARTESIAN_POINT('Origin',(79.6810800800795,7.105427357601E-15,96.4785797801185));
#182603=CARTESIAN_POINT('',(84.1408729574633,4.93000669486556,93.1536314377501));
#182604=CARTESIAN_POINT('',(84.661817490464,4.93000669486556,96.1080546967868));
#182605=CARTESIAN_POINT('',(85.5062788838804,-2.93305265169616,92.9128735333036));
#182606=CARTESIAN_POINT('Origin',(79.2469596359123,7.105427357601E-15,94.016560397588));
#182607=CARTESIAN_POINT('',(85.9403993280477,-2.93305265169627,95.3748929158341));
#182608=CARTESIAN_POINT('',(86.0272234168811,-2.93305265169616,95.8672967923402));
#182609=CARTESIAN_POINT('Origin',(79.6810800800795,7.105427357601E-15,96.4785797801185));
#182610=CARTESIAN_POINT('Origin',(79.6810800800795,7.105427357601E-15,96.4785797801185));
#182611=CARTESIAN_POINT('',(84.8261737214021,3.98351688341827,96.0790742588248));
#182612=CARTESIAN_POINT('',(73.672941151883,1.98656284024889,98.0456900829471));
#182613=CARTESIAN_POINT('Origin',(79.767904168913,7.105427357601E-15,96.9709836566246));
#182614=CARTESIAN_POINT('Ctrl Pts',(84.8261737218292,3.98351688369324,96.0790742592051));
#182615=CARTESIAN_POINT('Ctrl Pts',(84.7893586077452,4.12739717890119,96.0163852530348));
#182616=CARTESIAN_POINT('Ctrl Pts',(84.7515513858236,4.27253790876338,95.949354543555));
#182617=CARTESIAN_POINT('Ctrl Pts',(84.7127017230961,4.41924001707104,95.8779910058261));
#182618=CARTESIAN_POINT('Ctrl Pts',(84.6731714183888,4.56851233079177,95.805377186468));
#182619=CARTESIAN_POINT('Ctrl Pts',(84.6325609344404,4.71940100607333,95.7282775447341));
#182620=CARTESIAN_POINT('Ctrl Pts',(84.5908237439362,4.87217012300172,95.6467002846453));
#182621=CARTESIAN_POINT('Ctrl Pts',(84.5855648573402,4.89141903390341,95.636421548716));
#182622=CARTESIAN_POINT('Ctrl Pts',(84.5802881016179,4.91069773355134,95.6260717228448));
#182623=CARTESIAN_POINT('Ctrl Pts',(84.5749934016305,4.93000669486555,95.6156508202806));
#182624=CARTESIAN_POINT('Ctrl Pts',(73.4217608321114,2.93305265169625,97.5822666444029));
#182625=CARTESIAN_POINT('Ctrl Pts',(73.5563352960282,2.44228015705305,97.8471329035571));
#182626=CARTESIAN_POINT('Ctrl Pts',(73.6729411519522,1.98656284058742,98.0456900836835));
#182627=CARTESIAN_POINT('Origin',(76.9027092374091,7.31897349866028E-15,
80.7216557319231));
#182628=CARTESIAN_POINT('',(77.4879453938384,-5.17024070331411,78.7906949060641));
#182629=CARTESIAN_POINT('Origin',(76.5901425176087,7.31897349866028E-15,
78.9490017765011));
#182630=CARTESIAN_POINT('',(77.8005121136389,-5.17024070331411,80.5633488614862));
#182631=CARTESIAN_POINT('',(77.8005121136389,-5.17024070331411,80.5633488614862));
#182632=CARTESIAN_POINT('Origin',(76.9027092374091,7.31897349866028E-15,
80.7216557319231));
#182633=CARTESIAN_POINT('Origin',(76.5901425176087,7.15881389286582E-15,
78.9490017765011));
#182634=CARTESIAN_POINT('',(79.8067669160619,-4.75889434981443,76.1478855621002));
#182635=CARTESIAN_POINT('Ctrl Pts',(77.3632014628439,-5.90884651834311,
77.3332369269199));
#182636=CARTESIAN_POINT('Ctrl Pts',(77.3506260636621,-5.91108956208624,
77.3351752289124));
#182637=CARTESIAN_POINT('Ctrl Pts',(77.3380432219561,-5.91329153709518,
77.3371133880793));
#182638=CARTESIAN_POINT('Ctrl Pts',(77.2788465225023,-5.92345162954785,
77.3462257796284));
#182639=CARTESIAN_POINT('Ctrl Pts',(77.2321445292669,-5.9308869101996,77.3533979555682));
#182640=CARTESIAN_POINT('Ctrl Pts',(77.0753511513317,-5.95390907536924,
77.3774304758976));
#182641=CARTESIAN_POINT('Ctrl Pts',(76.9649056251977,-5.9669307645459,77.3942823635277));
#182642=CARTESIAN_POINT('Ctrl Pts',(76.6618859723424,-5.99395217460897,
77.4404025166063));
#182643=CARTESIAN_POINT('Ctrl Pts',(76.4688807497412,-6.00159982251535,
77.4696551679202));
#182644=CARTESIAN_POINT('Ctrl Pts',(75.9898225965994,-5.99694049464808,
77.5423125383788));
#182645=CARTESIAN_POINT('Ctrl Pts',(75.7043666432232,-5.97324907454268,
77.5856654911142));
#182646=CARTESIAN_POINT('Ctrl Pts',(75.3230929585664,-5.91332269699863,
77.6439595581747));
#182647=CARTESIAN_POINT('Ctrl Pts',(75.2248337194123,-5.8952978858626,77.6590155272321));
#182648=CARTESIAN_POINT('Ctrl Pts',(75.0561701016533,-5.85988616248508,
77.684917889718));
#182649=CARTESIAN_POINT('Ctrl Pts',(74.9855423687038,-5.84368697446087,
77.6957823251515));
#182650=CARTESIAN_POINT('Ctrl Pts',(74.8372974880923,-5.80678452955541,
77.7186216711591));
#182651=CARTESIAN_POINT('Ctrl Pts',(74.7597673880015,-5.78578732540409,
77.7305870417884));
#182652=CARTESIAN_POINT('Ctrl Pts',(74.5352351900356,-5.72000753864354,
77.7652901398945));
#182653=CARTESIAN_POINT('Ctrl Pts',(74.389509133096,-5.67103491114391,77.7878786138494));
#182654=CARTESIAN_POINT('Ctrl Pts',(74.0177569941561,-5.52966843690258,
77.8455618419822));
#182655=CARTESIAN_POINT('Ctrl Pts',(73.7951963689168,-5.42880121446908,
77.8801607875621));
#182656=CARTESIAN_POINT('Ctrl Pts',(73.4255301441766,-5.23281058087107,
77.9372382592266));
#182657=CARTESIAN_POINT('Ctrl Pts',(73.2752940405537,-5.14445614402073,
77.9603122637607));
#182658=CARTESIAN_POINT('Ctrl Pts',(73.0802293981269,-5.0178726511131,77.9899098159128));
#182659=CARTESIAN_POINT('Ctrl Pts',(73.0318522668943,-4.98546007820204,
77.9972189074484));
#182660=CARTESIAN_POINT('Ctrl Pts',(72.9498300101684,-4.92874514196303,
78.0095469802084));
#182661=CARTESIAN_POINT('Ctrl Pts',(72.915955360544,-4.90479576543907,78.0146186542405));
#182662=CARTESIAN_POINT('Ctrl Pts',(72.836423503911,-4.84731282746839,78.0264783303979));
#182663=CARTESIAN_POINT('Ctrl Pts',(72.7909846540467,-4.81347588462272,
78.03321724325));
#182664=CARTESIAN_POINT('Ctrl Pts',(72.5809447832021,-4.65236574538632,
78.0642156668819));
#182665=CARTESIAN_POINT('Ctrl Pts',(72.4224651225121,-4.51709693169309,
78.0871660182166));
#182666=CARTESIAN_POINT('Ctrl Pts',(72.0296418436112,-4.14463632815574,
78.1433767271642));
#182667=CARTESIAN_POINT('Ctrl Pts',(71.8072999109357,-3.89551556024683,
78.1745250907942));
#182668=CARTESIAN_POINT('Ctrl Pts',(71.5513795944523,-3.5555689415051,78.2099820159938));
#182669=CARTESIAN_POINT('Ctrl Pts',(71.4977899533019,-3.48087799896882,
78.2173775353426));
#182670=CARTESIAN_POINT('Ctrl Pts',(71.4051153999581,-3.34525020110468,
78.2301158055585));
#182671=CARTESIAN_POINT('Ctrl Pts',(71.3653820729729,-3.28478818682766,
78.2355588725799));
#182672=CARTESIAN_POINT('Ctrl Pts',(71.2813539430398,-3.15175759703652,
78.2470274246441));
#182673=CARTESIAN_POINT('Ctrl Pts',(71.2374838575667,-3.07893390829918,
78.2529873714572));
#182674=CARTESIAN_POINT('Ctrl Pts',(71.1048247433324,-2.84779572722359,
78.2709097487272));
#182675=CARTESIAN_POINT('Ctrl Pts',(71.0216063385146,-2.68633845119482,
78.2820050938437));
#182676=CARTESIAN_POINT('Ctrl Pts',(70.8091330343852,-2.22411028493838,
78.3096974484067));
#182677=CARTESIAN_POINT('Ctrl Pts',(70.6967675289738,-1.91613684032428,
78.3235569903442));
#182678=CARTESIAN_POINT('Ctrl Pts',(70.5766394231886,-1.48087712938312,
78.3360310584553));
#182679=CARTESIAN_POINT('Ctrl Pts',(70.5472829598692,-1.36027592592621,
78.3387604631571));
#182680=CARTESIAN_POINT('Ctrl Pts',(70.5113396586785,-1.19025983035946,
78.3415245968309));
#182681=CARTESIAN_POINT('Ctrl Pts',(70.5016583997892,-1.14154227312012,
78.3421934823646));
#182682=CARTESIAN_POINT('Ctrl Pts',(70.4855292057251,-1.05487694172736,
78.3431589091541));
#182683=CARTESIAN_POINT('Ctrl Pts',(70.4788445963702,-1.01697766904155,
78.3435049055603));
#182684=CARTESIAN_POINT('Ctrl Pts',(70.4637261463444,-0.926274313297555,
78.3441515691997));
#182685=CARTESIAN_POINT('Ctrl Pts',(70.455625741196,-0.873418202764558,
78.3443827825314));
#182686=CARTESIAN_POINT('Ctrl Pts',(70.4250964594316,-0.655148517543934,
78.3447546257627));
#182687=CARTESIAN_POINT('Ctrl Pts',(70.4087458166207,-0.48895652997662,
78.34366374263));
#182688=CARTESIAN_POINT('Ctrl Pts',(70.3798662879664,0.0166250587345677,
78.3365136485946));
#182689=CARTESIAN_POINT('Ctrl Pts',(70.3888296273098,0.356518233400312,
78.326530536891));
#182690=CARTESIAN_POINT('Ctrl Pts',(70.4415658323201,0.833400722205972,
78.3059594061294));
#182691=CARTESIAN_POINT('Ctrl Pts',(70.4618608837099,0.972495747144222,
78.2991498327544));
#182692=CARTESIAN_POINT('Ctrl Pts',(70.5011356182525,1.18873727561341,78.2873061484214));
#182693=CARTESIAN_POINT('Ctrl Pts',(70.5168337837154,1.26645557188026,78.2827915143711));
#182694=CARTESIAN_POINT('Ctrl Pts',(70.5500690224069,1.41581376705768,78.273614099924));
#182695=CARTESIAN_POINT('Ctrl Pts',(70.5673989816729,1.48748708892914,78.2689843157469));
#182696=CARTESIAN_POINT('Ctrl Pts',(70.6128044119319,1.66129737124357,78.2571996893161));
#182697=CARTESIAN_POINT('Ctrl Pts',(70.642258742329,1.76303311942229,78.2498276593441));
#182698=CARTESIAN_POINT('Ctrl Pts',(70.6949391624486,1.92857311319152,78.2370314251777));
#182699=CARTESIAN_POINT('Ctrl Pts',(70.7166006604831,1.9928695374001,78.2318590157327));
#182700=CARTESIAN_POINT('Ctrl Pts',(70.8094864699728,2.25394775023938,78.2100092635616));
#182701=CARTESIAN_POINT('Ctrl Pts',(70.8898007168674,2.44721072860713,78.1918547977842));
#182702=CARTESIAN_POINT('Ctrl Pts',(71.0747122441781,2.83410173331591,78.1510290794821));
#182703=CARTESIAN_POINT('Ctrl Pts',(71.1802104402173,3.0269305080173,78.1282031026571));
#182704=CARTESIAN_POINT('Ctrl Pts',(71.3292924509109,3.26722079926652,78.0961262804633));
#182705=CARTESIAN_POINT('Ctrl Pts',(71.3635404686114,3.32052102532757,78.0887675174631));
#182706=CARTESIAN_POINT('Ctrl Pts',(71.4217690184604,3.40806744445403,78.0762596672505));
#182707=CARTESIAN_POINT('Ctrl Pts',(71.4452824694775,3.44263164095962,78.0712093974405));
#182708=CARTESIAN_POINT('Ctrl Pts',(71.4993108488769,3.52029558856277,78.0596037690665));
#182709=CARTESIAN_POINT('Ctrl Pts',(71.5300341330659,3.56323833170345,78.0530043439425));
#182710=CARTESIAN_POINT('Ctrl Pts',(71.6461020388339,3.72101862213893,78.0280875790888));
#182711=CARTESIAN_POINT('Ctrl Pts',(71.7349337633283,3.83311675573491,78.0090475772363));
#182712=CARTESIAN_POINT('Ctrl Pts',(72.0518191055356,4.2047051751801,77.9414605108095));
#182713=CARTESIAN_POINT('Ctrl Pts',(72.2980985427034,4.44711785572191,77.8895214891883));
#182714=CARTESIAN_POINT('Ctrl Pts',(72.6559002459519,4.74230537440079,77.8155831897031));
#182715=CARTESIAN_POINT('Ctrl Pts',(72.7502668035142,4.81544297399608,77.7962031870972));
#182716=CARTESIAN_POINT('Ctrl Pts',(72.9074560487902,4.92977041751769,77.7641243732399));
#182717=CARTESIAN_POINT('Ctrl Pts',(72.9689814971273,4.97273749254529,77.7516164529573));
#182718=CARTESIAN_POINT('Ctrl Pts',(73.0936312062421,5.05627187149365,77.7263700008674));
#182719=CARTESIAN_POINT('Ctrl Pts',(73.156744392514,5.09683099428538,77.7136337322795));
#182720=CARTESIAN_POINT('Ctrl Pts',(73.3214067522893,5.19822833535625,77.6805191138512));
#182721=CARTESIAN_POINT('Ctrl Pts',(73.4240327992625,5.25720186420739,77.659990011575));
#182722=CARTESIAN_POINT('Ctrl Pts',(73.6606155811364,5.38374880961076,77.6128761954652));
#182723=CARTESIAN_POINT('Ctrl Pts',(73.7955091067059,5.44934283602376,77.5861614370359));
#182724=CARTESIAN_POINT('Ctrl Pts',(74.140470117322,5.60092360028518,77.5180840535909));
#182725=CARTESIAN_POINT('Ctrl Pts',(74.3532445281378,5.67993183846909,77.4763128793733));
#182726=CARTESIAN_POINT('Ctrl Pts',(74.7203187609538,5.79230262124935,77.4041621495857));
#182727=CARTESIAN_POINT('Ctrl Pts',(74.8724353469321,5.83218901281933,77.3742355919039));
#182728=CARTESIAN_POINT('Ctrl Pts',(75.0722053480645,5.87598185418345,77.3347496705309));
#182729=CARTESIAN_POINT('Ctrl Pts',(75.1186194837403,5.88556141947755,77.3255627041334));
#182730=CARTESIAN_POINT('Ctrl Pts',(75.2025522413787,5.90181368406663,77.308920105476));
#182731=CARTESIAN_POINT('Ctrl Pts',(75.24003145447,5.90868791565307,77.301477788033));
#182732=CARTESIAN_POINT('Ctrl Pts',(75.3235256948871,5.92315162420742,77.2848720637462));
#182733=CARTESIAN_POINT('Ctrl Pts',(75.3695672465983,5.93055540832166,77.2756983035838));
#182734=CARTESIAN_POINT('Ctrl Pts',(75.5226945858303,5.95328362363035,77.2451414975433));
#182735=CARTESIAN_POINT('Ctrl Pts',(75.6300968331472,5.96615666075899,77.2236346384187));
#182736=CARTESIAN_POINT('Ctrl Pts',(75.9218011656577,5.99283711972101,77.1651094690613));
#182737=CARTESIAN_POINT('Ctrl Pts',(76.1064794439842,6.00082178650795,77.1279387445323));
#182738=CARTESIAN_POINT('Ctrl Pts',(76.5850612752272,5.99852002942558,77.0316465318224));
#182739=CARTESIAN_POINT('Ctrl Pts',(76.8784014654325,5.97466202938466,76.9726769545909));
#182740=CARTESIAN_POINT('Ctrl Pts',(77.2664482155399,5.91305785057169,76.8950884073305));
#182741=CARTESIAN_POINT('Ctrl Pts',(77.3636815927662,5.89505524682198,76.8756798841097));
#182742=CARTESIAN_POINT('Ctrl Pts',(77.5307533009132,5.85967239758531,76.8423898515985));
#182743=CARTESIAN_POINT('Ctrl Pts',(77.6008057072906,5.84346835431527,76.8284494608582));
#182744=CARTESIAN_POINT('Ctrl Pts',(77.7479925249043,5.80652352441267,76.7991949427111));
#182745=CARTESIAN_POINT('Ctrl Pts',(77.8250405021964,5.78548336087124,76.783901965347));
#182746=CARTESIAN_POINT('Ctrl Pts',(78.0487572363214,5.71939886286866,76.7395484291761));
#182747=CARTESIAN_POINT('Ctrl Pts',(78.1941581527879,5.67010858638246,76.7107881629974));
#182748=CARTESIAN_POINT('Ctrl Pts',(78.5663566420792,5.52727369620649,76.6372268322258));
#182749=CARTESIAN_POINT('Ctrl Pts',(78.7896214687844,5.42500736946267,76.5931669259759));
#182750=CARTESIAN_POINT('Ctrl Pts',(79.160632137667,5.22586915268047,76.5195382731795));
#182751=CARTESIAN_POINT('Ctrl Pts',(79.3115795691863,5.13586652517762,76.4894516652793));
#182752=CARTESIAN_POINT('Ctrl Pts',(79.5038555214824,5.00914213561933,76.4507513777024));
#182753=CARTESIAN_POINT('Ctrl Pts',(79.5489743655254,4.97849234524775,76.441641459805));
#182754=CARTESIAN_POINT('Ctrl Pts',(79.6274610622036,4.92355615436399,76.4257345869609));
#182755=CARTESIAN_POINT('Ctrl Pts',(79.6610090100303,4.8995421684983,76.4189152439638));
#182756=CARTESIAN_POINT('Ctrl Pts',(79.7416892754808,4.84049101512612,76.4024663000907));
#182757=CARTESIAN_POINT('Ctrl Pts',(79.7885578906264,4.80509302272123,76.3928705667529));
#182758=CARTESIAN_POINT('Ctrl Pts',(79.8916332410604,4.72478546413949,76.3716886627046));
#182759=CARTESIAN_POINT('Ctrl Pts',(79.9475670358848,4.67953047094111,76.360140774091));
#182760=CARTESIAN_POINT('Ctrl Pts',(80.1271121698391,4.52872849850527,76.3229253994331));
#182761=CARTESIAN_POINT('Ctrl Pts',(80.2472493340549,4.41902999173157,76.2977918688098));
#182762=CARTESIAN_POINT('Ctrl Pts',(80.5696849700015,4.09923023111786,76.2299111378373));
#182763=CARTESIAN_POINT('Ctrl Pts',(80.7614230962109,3.87874331358182,76.1890571508917));
#182764=CARTESIAN_POINT('Ctrl Pts',(80.9927935034548,3.56951527749707,76.1394227644377));
#182765=CARTESIAN_POINT('Ctrl Pts',(81.0473347237524,3.49292103560964,76.1276911222302));
#182766=CARTESIAN_POINT('Ctrl Pts',(81.1405709663592,3.35523550989101,76.107582479175));
#182767=CARTESIAN_POINT('Ctrl Pts',(81.1799975354418,3.29468449084741,76.0990605515274));
#182768=CARTESIAN_POINT('Ctrl Pts',(81.2623716164879,3.16303589907158,76.0812131678088));
#182769=CARTESIAN_POINT('Ctrl Pts',(81.3049619008457,3.09172341205876,76.0719586563723));
#182770=CARTESIAN_POINT('Ctrl Pts',(81.4292432532612,2.87348182997442,76.044860509596));
#182771=CARTESIAN_POINT('Ctrl Pts',(81.5063177107551,2.72391007910021,76.0279273419392));
#182772=CARTESIAN_POINT('Ctrl Pts',(81.6927602095248,2.32160531003179,75.9864652001521));
#182773=CARTESIAN_POINT('Ctrl Pts',(81.7913600207955,2.06412738630946,75.9639957786357));
#182774=CARTESIAN_POINT('Ctrl Pts',(81.9249316956424,1.62823816926073,75.9318082406385));
#182775=CARTESIAN_POINT('Ctrl Pts',(81.9700452684845,1.45350869865743,75.9203794176626));
#182776=CARTESIAN_POINT('Ctrl Pts',(82.0187776624722,1.22248114638955,75.9069646256192));
#182777=CARTESIAN_POINT('Ctrl Pts',(82.0295164684856,1.16784487494401,75.9039140647558));
#182778=CARTESIAN_POINT('Ctrl Pts',(82.0464149938574,1.07511273889118,75.8989335929142));
#182779=CARTESIAN_POINT('Ctrl Pts',(82.0529673022251,1.03709562752515,75.8969472069984));
#182780=CARTESIAN_POINT('Ctrl Pts',(82.066971480648,0.950918421918528,75.8925681038923));
#182781=CARTESIAN_POINT('Ctrl Pts',(82.0742060528834,0.902725105582203,
75.8902069326183));
#182782=CARTESIAN_POINT('Ctrl Pts',(82.0971797447513,0.735989630105551,
75.8823506794407));
#182783=CARTESIAN_POINT('Ctrl Pts',(82.1099904223252,0.617051596595321,
75.8772911226832));
#182784=CARTESIAN_POINT('Ctrl Pts',(82.1363147537706,0.279113023273343,
75.8645656645264));
#182785=CARTESIAN_POINT('Ctrl Pts',(82.1414933687785,0.0596010719977289,
75.8582576433233));
#182786=CARTESIAN_POINT('Ctrl Pts',(82.1271196127539,-0.413320012160215,
75.8492799132833));
#182787=CARTESIAN_POINT('Ctrl Pts',(82.1035997858041,-0.666205737284208,
75.8473448774582));
#182788=CARTESIAN_POINT('Ctrl Pts',(82.0487369542072,-1.01733616280022,
75.8488792407423));
#182789=CARTESIAN_POINT('Ctrl Pts',(82.0305389796217,-1.11737104404053,
75.8498024922732));
#182790=CARTESIAN_POINT('Ctrl Pts',(81.99493222973,-1.28870363351042,75.8522258344588));
#182791=CARTESIAN_POINT('Ctrl Pts',(81.9787186485675,-1.36022969830393,
75.8534933047212));
#182792=CARTESIAN_POINT('Ctrl Pts',(81.941917219994,-1.51001194890346,75.8566852883709));
#182793=CARTESIAN_POINT('Ctrl Pts',(81.9210543179682,-1.58818430196483,
75.8586638568195));
#182794=CARTESIAN_POINT('Ctrl Pts',(81.856190435138,-1.81316741604527,75.8652583773005));
#182795=CARTESIAN_POINT('Ctrl Pts',(81.8082105628448,-1.95874004854391,
75.8706492320269));
#182796=CARTESIAN_POINT('Ctrl Pts',(81.6711855215464,-2.32709193130458,
75.8871040486295));
#182797=CARTESIAN_POINT('Ctrl Pts',(81.5743894861488,-2.54662762678099,
75.8996428677812));
#182798=CARTESIAN_POINT('Ctrl Pts',(81.3847491872626,-2.91570447120974,
75.9251142739667));
#182799=CARTESIAN_POINT('Ctrl Pts',(81.2978939989466,-3.06805259948355,
75.937024633462));
#182800=CARTESIAN_POINT('Ctrl Pts',(81.1709742064106,-3.26967982502136,
75.9545410210959));
#182801=CARTESIAN_POINT('Ctrl Pts',(81.1365636227905,-3.32248553230666,
75.9592997389913));
#182802=CARTESIAN_POINT('Ctrl Pts',(81.07789208696,-3.40949631070709,75.9674168694879));
#182803=CARTESIAN_POINT('Ctrl Pts',(81.0540897440679,-3.44400996024434,
75.9707103972316));
#182804=CARTESIAN_POINT('Ctrl Pts',(80.9991535597465,-3.52190824564898,
75.9783106934124));
#182805=CARTESIAN_POINT('Ctrl Pts',(80.9678002885372,-3.56512955816831,
75.9826485134425));
#182806=CARTESIAN_POINT('Ctrl Pts',(80.8475726083012,-3.72629742944358,
75.9992977067868));
#182807=CARTESIAN_POINT('Ctrl Pts',(80.7549573052134,-3.84133200312724,
76.0121547757447));
#182808=CARTESIAN_POINT('Ctrl Pts',(80.4011471605722,-4.24904527589804,
76.0616512699248));
#182809=CARTESIAN_POINT('Ctrl Pts',(80.1159069052643,-4.51904987235405,
76.1023284270222));
#182810=CARTESIAN_POINT('Ctrl Pts',(79.8067669160617,-4.75889434981455,
76.1478855621002));
#182811=CARTESIAN_POINT('',(81.8428871748401,-1.8061545077823,75.7888626245105));
#182812=CARTESIAN_POINT('Origin',(76.2081165267415,7.15881389286582E-15,
76.7824247198743));
#182813=CARTESIAN_POINT('Ctrl Pts',(81.8428871748402,-1.80615450778233,
75.7888626245105));
#182814=CARTESIAN_POINT('Ctrl Pts',(81.8719591200265,-1.71384756498248,
75.7859369317609));
#182815=CARTESIAN_POINT('Ctrl Pts',(81.8988209402735,-1.62084823720603,
75.783363797681));
#182816=CARTESIAN_POINT('Ctrl Pts',(81.9414678617161,-1.45874647804823,
75.7795189822176));
#182817=CARTESIAN_POINT('Ctrl Pts',(81.9582877020607,-1.38994087930884,
75.7780837356329));
#182818=CARTESIAN_POINT('Ctrl Pts',(81.9919918961584,-1.24079612489533,
75.7753965271836));
#182819=CARTESIAN_POINT('Ctrl Pts',(82.0084588570063,-1.16037622702758,
75.7742100949194));
#182820=CARTESIAN_POINT('Ctrl Pts',(82.0502944111701,-0.932667162109909,
75.7715953418392));
#182821=CARTESIAN_POINT('Ctrl Pts',(82.0718649456886,-0.784736073153573,
75.7707670718751));
#182822=CARTESIAN_POINT('Ctrl Pts',(82.1248190677507,-0.296004956785859,
75.7709825018011));
#182823=CARTESIAN_POINT('Ctrl Pts',(82.1328882059776,0.0466209745666767,
75.7757830109125));
#182824=CARTESIAN_POINT('Ctrl Pts',(82.1032487033638,0.536187394768259,
75.7903772288093));
#182825=CARTESIAN_POINT('Ctrl Pts',(82.0888706662041,0.683984223392767,
75.7958101691392));
#182826=CARTESIAN_POINT('Ctrl Pts',(82.0622311512114,0.882500704085245,
75.8046183533348));
#182827=CARTESIAN_POINT('Ctrl Pts',(82.054674676326,0.933839851342049,75.8070339409384));
#182828=CARTESIAN_POINT('Ctrl Pts',(82.0403903414168,1.02299497322353,75.8114760667689));
#182829=CARTESIAN_POINT('Ctrl Pts',(82.0339575547002,1.06085711266835,75.8134409606314));
#182830=CARTESIAN_POINT('Ctrl Pts',(82.0181600449413,1.14880983024054,75.8181884159474));
#182831=CARTESIAN_POINT('Ctrl Pts',(82.0085252681318,1.19884487504578,75.8210272401984));
#182832=CARTESIAN_POINT('Ctrl Pts',(81.9714478062439,1.37919586364177,75.8317477580379));
#182833=CARTESIAN_POINT('Ctrl Pts',(81.9403737538009,1.50868227430673,75.8403693110471));
#182834=CARTESIAN_POINT('Ctrl Pts',(81.8433187776311,1.86158388404592,75.8662781775486));
#182835=CARTESIAN_POINT('Ctrl Pts',(81.7687221410804,2.08226963852465,75.8851850182932));
#182836=CARTESIAN_POINT('Ctrl Pts',(81.6116193328735,2.47131842309215,75.9230950963684));
#182837=CARTESIAN_POINT('Ctrl Pts',(81.5336133417445,2.64124781514955,75.9413344553659));
#182838=CARTESIAN_POINT('Ctrl Pts',(81.394729232647,2.90996236340653,75.9728640143506));
#182839=CARTESIAN_POINT('Ctrl Pts',(81.3386481307373,3.01117114244377,75.9853929419478));
#182840=CARTESIAN_POINT('Ctrl Pts',(81.2414477063021,3.17518445276843,76.0067862102487));
#182841=CARTESIAN_POINT('Ctrl Pts',(81.2020008151637,3.23897707256013,76.0153902214272));
#182842=CARTESIAN_POINT('Ctrl Pts',(81.1200795984946,3.36604487126458,76.0331079746245));
#182843=CARTESIAN_POINT('Ctrl Pts',(81.0775737603586,3.42928237584866,76.0422261208518));
#182844=CARTESIAN_POINT('Ctrl Pts',(80.9626061256834,3.59344072359707,76.0667036341991));
#182845=CARTESIAN_POINT('Ctrl Pts',(80.8882011516666,3.69290889956414,76.0823626843461));
#182846=CARTESIAN_POINT('Ctrl Pts',(80.6130650129921,4.03768555344912,76.1397170584641));
#182847=CARTESIAN_POINT('Ctrl Pts',(80.3961140625166,4.26891458069115,76.1839440755937));
#182848=CARTESIAN_POINT('Ctrl Pts',(80.0436117577074,4.58900749139795,76.255380878693));
#182849=CARTESIAN_POINT('Ctrl Pts',(79.920897396206,4.69166634996503,76.280189675214));
#182850=CARTESIAN_POINT('Ctrl Pts',(79.7515027263841,4.82206715821595,76.3145137516457));
#182851=CARTESIAN_POINT('Ctrl Pts',(79.7082905702292,4.8543971396338,76.3232763498851));
#182852=CARTESIAN_POINT('Ctrl Pts',(79.6311903049683,4.91044715210589,76.3389310648733));
#182853=CARTESIAN_POINT('Ctrl Pts',(79.5974802293685,4.93441508779282,76.3457829725679));
#182854=CARTESIAN_POINT('Ctrl Pts',(79.5218274625517,4.98701329821702,76.361175204221));
#182855=CARTESIAN_POINT('Ctrl Pts',(79.4797651296251,5.01545681278895,76.3697426672664));
#182856=CARTESIAN_POINT('Ctrl Pts',(79.3002442708058,5.13349170842509,76.4063335220491));
#182857=CARTESIAN_POINT('Ctrl Pts',(79.1595328922465,5.21777990329696,76.4350738233895));
#182858=CARTESIAN_POINT('Ctrl Pts',(78.7944474871663,5.41611206244016,76.5095290878208));
#182859=CARTESIAN_POINT('Ctrl Pts',(78.5660108502608,5.52169887877698,76.5560039856362));
#182860=CARTESIAN_POINT('Ctrl Pts',(78.186723520633,5.66798482125429,76.6325975572483));
#182861=CARTESIAN_POINT('Ctrl Pts',(78.0397052596335,5.71800865899628,76.6621582554536));
#182862=CARTESIAN_POINT('Ctrl Pts',(77.8140839918658,5.78479494632151,76.7072965901127));
#182863=CARTESIAN_POINT('Ctrl Pts',(77.7368192802543,5.8059330580852,76.7227154060273));
#182864=CARTESIAN_POINT('Ctrl Pts',(77.5894755964486,5.84297486225297,76.7520450604194));
#182865=CARTESIAN_POINT('Ctrl Pts',(77.5194883824299,5.85919028039403,76.7659452401102));
#182866=CARTESIAN_POINT('Ctrl Pts',(77.3530083503173,5.89450921836859,76.7989390410556));
#182867=CARTESIAN_POINT('Ctrl Pts',(77.256297925221,5.91246240871852,76.8180495583339));
#182868=CARTESIAN_POINT('Ctrl Pts',(76.7884656538769,5.98702227382939,76.9102605580226));
#182869=CARTESIAN_POINT('Ctrl Pts',(76.4129196105907,6.00985752920379,76.9835054943814));
#182870=CARTESIAN_POINT('Ctrl Pts',(75.904700495134,5.99126318801624,77.0828782420069));
#182871=CARTESIAN_POINT('Ctrl Pts',(75.771767669737,5.98179104230586,77.1089021860041));
#182872=CARTESIAN_POINT('Ctrl Pts',(75.5509353441074,5.95836103982866,77.1522968390795));
#182873=CARTESIAN_POINT('Ctrl Pts',(75.4628157142397,5.94695194115564,77.1696566124335));
#182874=CARTESIAN_POINT('Ctrl Pts',(75.3318495589169,5.92691525344628,77.1955554370579));
#182875=CARTESIAN_POINT('Ctrl Pts',(75.2887800430601,5.91982575875605,77.2040884920697));
#182876=CARTESIAN_POINT('Ctrl Pts',(75.2078065139503,5.90555294357244,77.2201664611838));
#182877=CARTESIAN_POINT('Ctrl Pts',(75.169886550822,5.89847674541259,77.2277108500253));
#182878=CARTESIAN_POINT('Ctrl Pts',(75.0704421201887,5.8788872767805,77.2475319267741));
#182879=CARTESIAN_POINT('Ctrl Pts',(75.0090448498644,5.86574995822574,77.259805687597));
#182880=CARTESIAN_POINT('Ctrl Pts',(74.6882691700557,5.79162882224948,77.3240859886824));
#182881=CARTESIAN_POINT('Ctrl Pts',(74.4330489335526,5.71375314748594,77.3757491470365));
#182882=CARTESIAN_POINT('Ctrl Pts',(73.9108641123216,5.51416832098742,77.4816962347188));
#182883=CARTESIAN_POINT('Ctrl Pts',(73.6458310683007,5.3892457266918,77.5356035375481));
#182884=CARTESIAN_POINT('Ctrl Pts',(73.3072122383926,5.19732746331094,77.6043330533111));
#182885=CARTESIAN_POINT('Ctrl Pts',(73.2246214523536,5.14778774217879,77.6210869910811));
#182886=CARTESIAN_POINT('Ctrl Pts',(73.0825611618591,5.05774457682096,77.6498866465396));
#182887=CARTESIAN_POINT('Ctrl Pts',(73.0225620910214,5.01815203667619,77.6620444395812));
#182888=CARTESIAN_POINT('Ctrl Pts',(72.895983527477,4.93124852791776,77.6876837107054));
#182889=CARTESIAN_POINT('Ctrl Pts',(72.8296260867835,4.88362757161157,77.7011188406143));
#182890=CARTESIAN_POINT('Ctrl Pts',(72.6321153230523,4.73556285251598,77.7411011869603));
#182891=CARTESIAN_POINT('Ctrl Pts',(72.5040920182839,4.63091085363375,77.7670055485619));
#182892=CARTESIAN_POINT('Ctrl Pts',(72.3289838485916,4.47506284305219,77.8025008632107));
#182893=CARTESIAN_POINT('Ctrl Pts',(72.2782280441991,4.42827291545422,77.8127978397302));
#182894=CARTESIAN_POINT('Ctrl Pts',(72.0623293565463,4.22214170727489,77.8566603970351));
#182895=CARTESIAN_POINT('Ctrl Pts',(71.9055440613095,4.05401419205986,77.8886679947361));
#182896=CARTESIAN_POINT('Ctrl Pts',(71.7044004765138,3.81150794798109,77.9303447454054));
#182897=CARTESIAN_POINT('Ctrl Pts',(71.6514310915522,3.74477867114699,77.9413865579926));
#182898=CARTESIAN_POINT('Ctrl Pts',(71.5597852808818,3.62408567351391,77.9606436757048));
#182899=CARTESIAN_POINT('Ctrl Pts',(71.5205492818374,3.57057870151534,77.9689417561));
#182900=CARTESIAN_POINT('Ctrl Pts',(71.4578667079739,3.48202676119671,77.9823026922628));
#182901=CARTESIAN_POINT('Ctrl Pts',(71.4338879269392,3.44737718493032,77.9874403431168));
#182902=CARTESIAN_POINT('Ctrl Pts',(71.3816229694524,3.37011238400974,77.9987015054357));
#182903=CARTESIAN_POINT('Ctrl Pts',(71.3535125235248,3.32737971828664,78.0047998540314));
#182904=CARTESIAN_POINT('Ctrl Pts',(71.2662696451409,3.19096399125769,78.0238495217737));
#182905=CARTESIAN_POINT('Ctrl Pts',(71.2091762194463,3.09596283196378,78.036501483874));
#182906=CARTESIAN_POINT('Ctrl Pts',(71.0379664607983,2.79227821644302,78.0749481162468));
#182907=CARTESIAN_POINT('Ctrl Pts',(70.9335308783647,2.57820490389664,78.0991683841703));
#182908=CARTESIAN_POINT('Ctrl Pts',(70.757100608402,2.15462571188343,78.1412735040649));
#182909=CARTESIAN_POINT('Ctrl Pts',(70.6834171712819,1.94626824508627,78.1594618326851));
#182910=CARTESIAN_POINT('Ctrl Pts',(70.5965129130708,1.64997726713302,78.181759359022));
#182911=CARTESIAN_POINT('Ctrl Pts',(70.5736320346361,1.56520715477846,78.1877443021302));
#182912=CARTESIAN_POINT('Ctrl Pts',(70.5352767090858,1.40980413738651,78.1980000643091));
#182913=CARTESIAN_POINT('Ctrl Pts',(70.5192115349662,1.33934191401665,78.2023858682363));
#182914=CARTESIAN_POINT('Ctrl Pts',(70.4859425970943,1.18041816187274,78.211688558623));
#182915=CARTESIAN_POINT('Ctrl Pts',(70.4694380299398,1.09182034121506,78.2164687191469));
#182916=CARTESIAN_POINT('Ctrl Pts',(70.4208886899886,0.794745074487697,
78.2311615562803));
#182917=CARTESIAN_POINT('Ctrl Pts',(70.3976831131773,0.584901259477872,
78.2393541283082));
#182918=CARTESIAN_POINT('Ctrl Pts',(70.3694861764948,0.101162741297917,
78.2535234503463));
#182919=CARTESIAN_POINT('Ctrl Pts',(70.371951631181,-0.172730905845747,
78.2581045926711));
#182920=CARTESIAN_POINT('Ctrl Pts',(70.4030275290813,-0.578271616274934,
78.2604392843645));
#182921=CARTESIAN_POINT('Ctrl Pts',(70.4175532912998,-0.710622889317259,
78.2604933345498));
#182922=CARTESIAN_POINT('Ctrl Pts',(70.4435634754622,-0.892259226385203,
78.2596788716901));
#182923=CARTESIAN_POINT('Ctrl Pts',(70.4513262536437,-0.942040066818519,
78.259362969781));
#182924=CARTESIAN_POINT('Ctrl Pts',(70.466113725168,-1.02967383407506,78.2586497579256));
#182925=CARTESIAN_POINT('Ctrl Pts',(70.4728799543504,-1.06756670307819,
78.2582897173655));
#182926=CARTESIAN_POINT('Ctrl Pts',(70.48994323149,-1.15812897158568,78.2573049861004));
#182927=CARTESIAN_POINT('Ctrl Pts',(70.5005796137709,-1.21072984648261,
78.2566312819108));
#182928=CARTESIAN_POINT('Ctrl Pts',(70.5462490698922,-1.42209918843184,
78.2534972905141));
#182929=CARTESIAN_POINT('Ctrl Pts',(70.5869606291509,-1.57955875111542,
78.2501860690012));
#182930=CARTESIAN_POINT('Ctrl Pts',(70.7184668646324,-2.01525440478615,
78.2379951539103));
#182931=CARTESIAN_POINT('Ctrl Pts',(70.8230993559022,-2.28878080897071,
78.2267782649833));
#182932=CARTESIAN_POINT('Ctrl Pts',(71.0203438686532,-2.71054483735033,
78.203093985243));
#182933=CARTESIAN_POINT('Ctrl Pts',(71.1004191817987,-2.8642613652786,78.1930106878791));
#182934=CARTESIAN_POINT('Ctrl Pts',(71.2288745573352,-3.0870245578603,78.1761591723132));
#182935=CARTESIAN_POINT('Ctrl Pts',(71.272325092367,-3.1588813259545,78.170360548172));
#182936=CARTESIAN_POINT('Ctrl Pts',(71.3560277230687,-3.29101901361857,
78.1590136893739));
#182937=CARTESIAN_POINT('Ctrl Pts',(71.3958988942966,-3.35152926486004,
78.1535404459856));
#182938=CARTESIAN_POINT('Ctrl Pts',(71.4896724508966,-3.48842304696753,
78.1405195282612));
#182939=CARTESIAN_POINT('Ctrl Pts',(71.5442729109051,-3.56429186663778,
78.132832846811));
#182940=CARTESIAN_POINT('Ctrl Pts',(71.7906540096913,-3.89038865240792,
78.0977307529199));
#182941=CARTESIAN_POINT('Ctrl Pts',(71.9999369287116,-4.12637041442099,
78.0668325506397));
#182942=CARTESIAN_POINT('Ctrl Pts',(72.3796812003209,-4.49198116248029,
78.0099984305344));
#182943=CARTESIAN_POINT('Ctrl Pts',(72.5404353036647,-4.631011607848,77.9857555140472));
#182944=CARTESIAN_POINT('Ctrl Pts',(72.7564840271555,-4.79851050232391,
77.9532751212576));
#182945=CARTESIAN_POINT('Ctrl Pts',(72.8053421584588,-4.83519606355928,
77.9459365106532));
#182946=CARTESIAN_POINT('Ctrl Pts',(72.8884135976851,-4.89558659048793,
77.9334815957941));
#182947=CARTESIAN_POINT('Ctrl Pts',(72.9223284084198,-4.91969992549469,
77.9284033245493));
#182948=CARTESIAN_POINT('Ctrl Pts',(73.0002989528576,-4.97390937553228,
77.9167450209659));
#182949=CARTESIAN_POINT('Ctrl Pts',(73.0445097027769,-5.00376947507537,
77.9101454846803));
#182950=CARTESIAN_POINT('Ctrl Pts',(73.2103579530749,-5.1125521989381,77.8854141938693));
#182951=CARTESIAN_POINT('Ctrl Pts',(73.3344442080653,-5.18757649789067,
77.8669599165302));
#182952=CARTESIAN_POINT('Ctrl Pts',(73.6698945540302,-5.37394192361085,
77.8170121825215));
#182953=CARTESIAN_POINT('Ctrl Pts',(73.8853873666549,-5.47712857415794,
77.7848589719973));
#182954=CARTESIAN_POINT('Ctrl Pts',(74.2782576057679,-5.63680376075511,
77.7257310415124));
#182955=CARTESIAN_POINT('Ctrl Pts',(74.4532461325465,-5.69848676943401,
77.6992283193579));
#182956=CARTESIAN_POINT('Ctrl Pts',(74.711371125651,-5.77599892194807,77.6598294477604));
#182957=CARTESIAN_POINT('Ctrl Pts',(74.7924675727333,-5.79846782118944,
77.6474094354249));
#182958=CARTESIAN_POINT('Ctrl Pts',(74.9435712038005,-5.8368637282888,77.6241894887138));
#182959=CARTESIAN_POINT('Ctrl Pts',(75.0134466410989,-5.85326368132142,
77.6134212609044));
#182960=CARTESIAN_POINT('Ctrl Pts',(75.1728585393736,-5.88761072186219,
77.5887880308129));
#182961=CARTESIAN_POINT('Ctrl Pts',(75.2625420519347,-5.90475683466136,
77.5748820450661));
#182962=CARTESIAN_POINT('Ctrl Pts',(75.7325036040162,-5.9832933221517,77.5017899383352));
#182963=CARTESIAN_POINT('Ctrl Pts',(76.1175034016835,-6.00918872011661,
77.4410845524726));
#182964=CARTESIAN_POINT('Ctrl Pts',(76.6422572293234,-5.99273176795224,
77.3585511041752));
#182965=CARTESIAN_POINT('Ctrl Pts',(76.7820434835449,-5.98332275946202,
77.3365946589979));
#182966=CARTESIAN_POINT('Ctrl Pts',(77.0128440490101,-5.95945447064461,
77.3005139876206));
#182967=CARTESIAN_POINT('Ctrl Pts',(77.1040797843196,-5.94784500323426,
77.2862962950022));
#182968=CARTESIAN_POINT('Ctrl Pts',(77.2389014114205,-5.92745907971508,
77.2653882840629));
#182969=CARTESIAN_POINT('Ctrl Pts',(77.2827078619588,-5.92032636533896,
77.258610896689));
#182970=CARTESIAN_POINT('Ctrl Pts',(77.3337116152199,-5.91142730893575,
77.2507420206451));
#182971=CARTESIAN_POINT('Ctrl Pts',(77.3409869335096,-5.91014377924753,
77.2496201062063));
#182972=CARTESIAN_POINT('Ctrl Pts',(77.3482598983342,-5.90884651798042,
77.2484990919142));
#182973=CARTESIAN_POINT('Origin',(76.5149506510185,7.15881389286582E-15,
78.5225675105249));
#182974=CARTESIAN_POINT('',(80.6284101054663,-3.63675684748494,78.0903820385128));
#182975=CARTESIAN_POINT('',(77.5109869441485,-5.49094931682848,78.5957139706103));
#182976=CARTESIAN_POINT('Ctrl Pts',(77.5109869441485,-5.49094931682847,
78.5957139706103));
#182977=CARTESIAN_POINT('Ctrl Pts',(78.1896918683254,-5.35556772975862,
78.4841869022237));
#182978=CARTESIAN_POINT('Ctrl Pts',(78.7554088112724,-5.1055662767554,78.393188160418));
#182979=CARTESIAN_POINT('Ctrl Pts',(79.7377353752645,-4.52841761382738,
78.234158897099));
#182980=CARTESIAN_POINT('Ctrl Pts',(80.2236625868063,-4.11908110158411,
78.1550172499348));
#182981=CARTESIAN_POINT('Ctrl Pts',(80.6284101060512,-3.63675684793529,
78.0903820388149));
#182982=CARTESIAN_POINT('',(81.5941173588847,2.04265365340621,77.9201017942693));
#182983=CARTESIAN_POINT('Origin',(76.5650785620786,7.15881389286582E-15,
78.8068570211757));
#182984=CARTESIAN_POINT('Origin',(22.3114963328544,145.306839242356,89.0571204175862));
#182985=CARTESIAN_POINT('Ctrl Pts',(79.5631824082928,5.13997981405092,77.9850820082628));
#182986=CARTESIAN_POINT('Ctrl Pts',(79.144532880795,5.38518891260996,78.0646192810899));
#182987=CARTESIAN_POINT('Ctrl Pts',(78.6966575569264,5.57679262082688,78.1497307045318));
#182988=CARTESIAN_POINT('Ctrl Pts',(77.8259665816532,5.82815848696469,78.3136925708069));
#182989=CARTESIAN_POINT('Ctrl Pts',(77.4081857473062,5.90127337120631,78.3917886262775));
#182990=CARTESIAN_POINT('Ctrl Pts',(76.5284259338047,5.95799929590254,78.5555726318262));
#182991=CARTESIAN_POINT('Ctrl Pts',(75.8630971584906,5.94870954755889,78.6785004071637));
#182992=CARTESIAN_POINT('Ctrl Pts',(74.3473318554912,5.52279212407711,78.9648707259658));
#182993=CARTESIAN_POINT('Ctrl Pts',(73.6512982737334,5.16369081654802,79.097653170836));
#182994=CARTESIAN_POINT('Ctrl Pts',(72.5306476584885,4.26987919295954,79.3103869139622));
#182995=CARTESIAN_POINT('Ctrl Pts',(72.0833704466692,3.77061895417284,79.3950648833961));
#182996=CARTESIAN_POINT('Ctrl Pts',(71.3290937718838,2.54917482922943,79.5447002438745));
#182997=CARTESIAN_POINT('Ctrl Pts',(71.0583979266505,1.81538535021859,79.6026474139665));
#182998=CARTESIAN_POINT('Ctrl Pts',(70.8269162740687,0.386676405105633,
79.6589560215703));
#182999=CARTESIAN_POINT('Ctrl Pts',(70.8324701147635,-0.296931580282131,
79.6638068701898));
#183000=CARTESIAN_POINT('Ctrl Pts',(71.0981688558512,-1.70847266736971,
79.6329869040131));
#183001=CARTESIAN_POINT('Ctrl Pts',(71.3889392755114,-2.42207361322268,
79.5923592140419));
#183002=CARTESIAN_POINT('Ctrl Pts',(72.1805383634408,-3.63125885150102,
79.4694000462425));
#183003=CARTESIAN_POINT('Ctrl Pts',(72.6575318459149,-4.13689966793945,
79.3916265768121));
#183004=CARTESIAN_POINT('Ctrl Pts',(73.8589324237686,-5.01033879056241,
79.1962536241068));
#183005=CARTESIAN_POINT('Ctrl Pts',(74.554062491525,-5.29847388859498,79.0841805175807));
#183006=CARTESIAN_POINT('Ctrl Pts',(75.8658885405282,-5.60208752807489,
78.8686428509867));
#183007=CARTESIAN_POINT('Ctrl Pts',(76.5406155618653,-5.63487017566596,
78.7559603591494));
#183008=CARTESIAN_POINT('Ctrl Pts',(77.3072788239429,-5.52853753302272,
78.6292461832499));
#183009=CARTESIAN_POINT('Ctrl Pts',(77.4103761181366,-5.51101820511365,
78.6122466788217));
#183010=CARTESIAN_POINT('Ctrl Pts',(77.5109869441485,-5.49094931682847,
78.5957139706103));
#183011=CARTESIAN_POINT('',(77.5410110809953,-5.90884651807327,78.3416453728827));
#183012=CARTESIAN_POINT('Origin',(76.1212924379081,7.14546725904962E-15,
76.2900208433682));
#183013=CARTESIAN_POINT('',(76.9605608422114,-4.33315411413756,76.6497484855763));
#183014=CARTESIAN_POINT('',(75.4556722114252,4.33315411325374,76.9151009541453));
#183015=CARTESIAN_POINT('Origin',(76.2081165267415,7.14546725904962E-15,
76.7824247198743));
#183016=CARTESIAN_POINT('',(76.0634408332593,4.33315411325374,80.361928089688));
#183017=CARTESIAN_POINT('',(75.3688481225918,4.33315411325374,76.4226970776392));
#183018=CARTESIAN_POINT('Origin',(76.8158851485756,7.14546725904962E-15,
80.229251855417));
#183019=CARTESIAN_POINT('Origin',(76.2081165267415,7.14546725904962E-15,
76.7824247198743));
#183020=CARTESIAN_POINT('Origin',(76.8158851485756,7.19646783916074E-15,
80.229251855417));
#183021=CARTESIAN_POINT('',(79.2648504730746,-0.865626271753975,80.3051464998313));
#183022=CARTESIAN_POINT('',(77.3387849203051,-2.51125977018251,80.6447638243076));
#183023=CARTESIAN_POINT('Origin',(76.9027092374091,7.19646783916074E-15,
80.7216557319231));
#183024=CARTESIAN_POINT('',(79.2648504730747,0.865626271753664,80.3051464998313));
#183025=CARTESIAN_POINT('Origin',(76.9027092374091,7.19646783916074E-15,
80.7216557319231));
#183026=CARTESIAN_POINT('',(82.0432213157451,0.865626271753682,96.0620705480267));
#183027=CARTESIAN_POINT('',(80.6540358944099,0.865626271753672,88.183608523929));
#183028=CARTESIAN_POINT('',(79.2450043973393,2.51125977018097,96.5554716886163));
#183029=CARTESIAN_POINT('Origin',(79.6810800800795,7.19646783916074E-15,
96.4785797801185));
#183030=CARTESIAN_POINT('',(82.043221315745,-0.865626271753956,96.0620705480267));
#183031=CARTESIAN_POINT('Origin',(79.6810800800795,7.19646783916074E-15,
96.4785797801185));
#183032=CARTESIAN_POINT('',(80.6540358944098,-0.865626271753965,88.1836085239291));
#183033=CARTESIAN_POINT('Origin',(79.6810800800795,7.19646783916074E-15,
96.4785797801185));
#183034=CARTESIAN_POINT('Ctrl Pts',(82.043221315745,0.865626271753621,96.0620705480265));
#183035=CARTESIAN_POINT('Ctrl Pts',(82.0992182044097,0.72751926106728,96.057947244922));
#183036=CARTESIAN_POINT('Ctrl Pts',(82.1409660117247,0.58564103397652,96.0548556380306));
#183037=CARTESIAN_POINT('Ctrl Pts',(82.2309139993029,0.128835088516363,
96.048187545496));
#183038=CARTESIAN_POINT('Ctrl Pts',(82.2265395302818,-0.219618264988888,
96.0485181512139));
#183039=CARTESIAN_POINT('Ctrl Pts',(82.1191291777162,-0.657108269115395,
96.0564710052956));
#183040=CARTESIAN_POINT('Ctrl Pts',(82.0847823537726,-0.763122885228353,
96.0590102216189));
#183041=CARTESIAN_POINT('Ctrl Pts',(82.0432213157448,-0.865626271754031,
96.0620705480265));
#183042=CARTESIAN_POINT('',(79.246323450496,3.00366364624538,97.0629524103545));
#183043=CARTESIAN_POINT('',(79.2450043973393,2.51125977018115,96.5554716886164));
#183044=CARTESIAN_POINT('Origin',(79.767904168913,7.19646783916074E-15,
96.9709836566246));
#183045=CARTESIAN_POINT('Origin',(76.8158851485756,7.19646783916074E-15,
80.229251855417));
#183046=CARTESIAN_POINT('Ctrl Pts',(79.2648504732428,-0.865626271722663,
80.3051465007115));
#183047=CARTESIAN_POINT('Ctrl Pts',(79.3741062412579,-0.586356325647426,
80.2742536009109));
#183048=CARTESIAN_POINT('Ctrl Pts',(79.4277739616774,-0.283930880250993,
80.2591373622784));
#183049=CARTESIAN_POINT('Ctrl Pts',(79.4277739616774,-7.39557098644699E-30,
80.2591373622784));
#183050=CARTESIAN_POINT('Ctrl Pts',(79.4277739616774,0.283930880250773,
80.2591373622784));
#183051=CARTESIAN_POINT('Ctrl Pts',(79.3741062412579,0.58635632564696,80.2742536009109));
#183052=CARTESIAN_POINT('Ctrl Pts',(79.2648504732431,0.86562627172201,80.3051465007115));
#183053=CARTESIAN_POINT('',(77.3374658671472,-3.00366364668724,80.1372831021155));
#183054=CARTESIAN_POINT('',(77.3374658671472,-3.00366364668724,80.1372831021155));
#183055=CARTESIAN_POINT('Origin',(76.8158851485756,7.19646783916074E-15,
80.229251855417));
#183056=CARTESIAN_POINT('Origin',(76.1212924379081,7.15881389286582E-15,
76.2900208433682));
#183057=CARTESIAN_POINT('Origin',(76.1212924379081,7.15881389286582E-15,
76.2900208433682));
#183058=CARTESIAN_POINT('',(77.1196285163625,-5.58066418896375,76.2833680310246));
#183059=CARTESIAN_POINT('Ctrl Pts',(77.1196277140212,-5.58095582281337,
76.283067472893));
#183060=CARTESIAN_POINT('Ctrl Pts',(76.9928283292005,-5.59398387932902,
76.2953436706019));
#183061=CARTESIAN_POINT('Ctrl Pts',(76.8409545289557,-5.60874287494297,
76.3141618693424));
#183062=CARTESIAN_POINT('Ctrl Pts',(76.5747214953194,-5.61991440458212,
76.3473866361007));
#183063=CARTESIAN_POINT('Ctrl Pts',(76.4795857142021,-5.62178133713042,
76.359292303505));
#183064=CARTESIAN_POINT('Ctrl Pts',(76.3528445946748,-5.6205988089503,76.3751832134439));
#183065=CARTESIAN_POINT('Ctrl Pts',(76.331876307243,-5.62025437321422,76.3778119200945));
#183066=CARTESIAN_POINT('Ctrl Pts',(76.2865965392702,-5.61926007964262,
76.3834857866538));
#183067=CARTESIAN_POINT('Ctrl Pts',(76.2191382964961,-5.61735584476887,
76.3919355893989));
#183068=CARTESIAN_POINT('Ctrl Pts',(76.1530768483827,-5.61426740474037,
76.4002001849428));
#183069=CARTESIAN_POINT('Ctrl Pts',(75.7623791796731,-5.59141776986316,
76.4490321459133));
#183070=CARTESIAN_POINT('Ctrl Pts',(75.455903832143,-5.54095283542196,76.4869797101295));
#183071=CARTESIAN_POINT('Ctrl Pts',(74.9267679368036,-5.41933799813517,
76.5515711076113));
#183072=CARTESIAN_POINT('Ctrl Pts',(74.7038794990428,-5.34810738982767,
76.5782551240242));
#183073=CARTESIAN_POINT('Ctrl Pts',(74.3361966660066,-5.21233203848455,
76.62132814975));
#183074=CARTESIAN_POINT('Ctrl Pts',(74.1912453772525,-5.14773003290795,
76.6377448236165));
#183075=CARTESIAN_POINT('Ctrl Pts',(74.0817004664548,-5.09516704230596,
76.6496559375717));
#183076=CARTESIAN_POINT('Ctrl Pts',(81.8428871744966,-1.80615450764722,
75.7888626250267));
#183077=CARTESIAN_POINT('Ctrl Pts',(81.7921281915313,-1.9400359292157,75.7901202345789));
#183078=CARTESIAN_POINT('Ctrl Pts',(81.736482277759,-2.07298945865901,75.7923157524007));
#183079=CARTESIAN_POINT('Ctrl Pts',(81.6758444736533,-2.20457874696473,
75.7954174203319));
#183080=CARTESIAN_POINT('Ctrl Pts',(81.6158044677516,-2.33487076137691,
75.7984885104488));
#183081=CARTESIAN_POINT('Ctrl Pts',(81.5508702154952,-2.46382504862596,
75.8024480243678));
#183082=CARTESIAN_POINT('Ctrl Pts',(81.4809800071083,-2.59098807599447,
75.8072580498469));
#183083=CARTESIAN_POINT('Ctrl Pts',(81.4121175334748,-2.71628117243014,
75.8119973439537));
#183084=CARTESIAN_POINT('Ctrl Pts',(81.3384435597397,-2.83983499752331,
75.8175623600099));
#183085=CARTESIAN_POINT('Ctrl Pts',(81.2599420646749,-2.96119065762395,
75.8239092506691));
#183086=CARTESIAN_POINT('Ctrl Pts',(81.2088340415657,-3.04019868002837,
75.8280413634933));
#183087=CARTESIAN_POINT('Ctrl Pts',(81.1556807075916,-3.11827448547332,
75.8325047261173));
#183088=CARTESIAN_POINT('Ctrl Pts',(81.1004883555888,-3.19528657070903,
75.8372853496264));
#183089=CARTESIAN_POINT('Ctrl Pts',(81.0027104922194,-3.33171991472714,
75.8457546236349));
#183090=CARTESIAN_POINT('Ctrl Pts',(80.8983883938494,-3.46483276372604,
75.8551462426669));
#183091=CARTESIAN_POINT('Ctrl Pts',(80.7877291090633,-3.59398652754898,
75.8655119707144));
#183092=CARTESIAN_POINT('Ctrl Pts',(80.677602856128,-3.72251817394275,75.8758277683542));
#183093=CARTESIAN_POINT('Ctrl Pts',(80.5612002832816,-3.84712861067232,
75.8871083198699));
#183094=CARTESIAN_POINT('Ctrl Pts',(80.4387761426652,-3.96719064408858,
75.899395708375));
#183095=CARTESIAN_POINT('Ctrl Pts',(80.3172662063421,-4.08635611228608,
75.9115913406033));
#183096=CARTESIAN_POINT('Ctrl Pts',(80.1898242819621,-4.20104068895251,
75.9247788317873));
#183097=CARTESIAN_POINT('Ctrl Pts',(80.0567498702629,-4.31063582828496,
75.9389904400899));
#183098=CARTESIAN_POINT('Ctrl Pts',(80.0274847959161,-4.33473745578535,
75.9421157875421));
#183099=CARTESIAN_POINT('Ctrl Pts',(79.9979475148131,-4.3585929681685,75.9452906295833));
#183100=CARTESIAN_POINT('Ctrl Pts',(79.9681415442571,-4.38219593621601,
75.9485152507764));
#183101=CARTESIAN_POINT('Ctrl Pts',(79.8517313649804,-4.47437967291755,
75.9611093292171));
#183102=CARTESIAN_POINT('Ctrl Pts',(79.7312463819954,-4.56269272089981,
75.9744637622036));
#183103=CARTESIAN_POINT('Ctrl Pts',(79.6069578462149,-4.64669689424489,
75.9885545936021));
#183104=CARTESIAN_POINT('Ctrl Pts',(79.4968333490383,-4.7211278728727,76.0010396205825));
#183105=CARTESIAN_POINT('Ctrl Pts',(79.3837235417294,-4.79217618243141,
76.0141026401752));
#183106=CARTESIAN_POINT('Ctrl Pts',(79.2678476526638,-4.85955146850915,
76.0277216023301));
#183107=CARTESIAN_POINT('Ctrl Pts',(79.1445198768333,-4.93125960593888,
76.0422163891682));
#183108=CARTESIAN_POINT('Ctrl Pts',(79.0180581340044,-4.99880154775553,
76.0573371091365));
#183109=CARTESIAN_POINT('Ctrl Pts',(78.8887553248201,-5.06182011558757,
76.0730252949464));
#183110=CARTESIAN_POINT('Ctrl Pts',(78.824103920228,-5.09332939950359,76.0808693878514));
#183111=CARTESIAN_POINT('Ctrl Pts',(78.7587427054292,-5.12370793042999,
76.0888549612484));
#183112=CARTESIAN_POINT('Ctrl Pts',(78.692710765976,-5.15291179036842,76.0969723772704));
#183113=CARTESIAN_POINT('Ctrl Pts',(78.6759572861809,-5.16032133007703,
76.0990319103757));
#183114=CARTESIAN_POINT('Ctrl Pts',(78.6574625598256,-5.16840084401436,
76.1013076781226));
#183115=CARTESIAN_POINT('Ctrl Pts',(78.6383605611387,-5.17660867914664,
76.1036565734103));
#183116=CARTESIAN_POINT('Ctrl Pts',(78.6198183797459,-5.18457596939512,
76.1059366302364));
#183117=CARTESIAN_POINT('Ctrl Pts',(78.6007039910472,-5.19266389923966,
76.1082855925168));
#183118=CARTESIAN_POINT('Ctrl Pts',(78.5820713772747,-5.20042139045395,
76.1105696052704));
#183119=CARTESIAN_POINT('Ctrl Pts',(78.5442436021413,-5.21617058360719,
76.1152065886747));
#183120=CARTESIAN_POINT('Ctrl Pts',(78.5068893167332,-5.23121722635507,
76.1197706818044));
#183121=CARTESIAN_POINT('Ctrl Pts',(78.4700318597412,-5.24559853331115,
76.1242565665862));
#183122=CARTESIAN_POINT('Ctrl Pts',(78.3883262999547,-5.27747899472131,
76.1342008697788));
#183123=CARTESIAN_POINT('Ctrl Pts',(78.3090658667927,-5.30608739681267,
76.1437570191419));
#183124=CARTESIAN_POINT('Ctrl Pts',(78.2324656107456,-5.33182355776652,
76.1528794079931));
#183125=CARTESIAN_POINT('Ctrl Pts',(78.1547737950188,-5.3579264610403,76.1621317916037));
#183126=CARTESIAN_POINT('Ctrl Pts',(78.0798181702974,-5.38107504391943,
76.1709380246403));
#183127=CARTESIAN_POINT('Ctrl Pts',(78.0077749223473,-5.40166281994532,
76.1792590199731));
#183128=CARTESIAN_POINT('Ctrl Pts',(77.9342932975165,-5.42266164047438,
76.1877461478395));
#183129=CARTESIAN_POINT('Ctrl Pts',(77.8638411785452,-5.44099673380601,
76.1957285260235));
#183130=CARTESIAN_POINT('Ctrl Pts',(77.7965607960489,-5.45705568395242,
76.2031725645302));
#183131=CARTESIAN_POINT('Ctrl Pts',(77.7601365449749,-5.46574967780942,
76.2072026178312));
#183132=CARTESIAN_POINT('Ctrl Pts',(77.724641169074,-5.4737760041616,76.2110750177584));
#183133=CARTESIAN_POINT('Ctrl Pts',(77.6900924558518,-5.48119208907128,
76.2147852774337));
#183134=CARTESIAN_POINT('Ctrl Pts',(77.6622650361554,-5.487165408713,76.2177737231249));
#183135=CARTESIAN_POINT('Ctrl Pts',(77.6350517701762,-5.49274348408649,
76.220657656134));
#183136=CARTESIAN_POINT('Ctrl Pts',(77.608460664494,-5.49795545559569,76.2234355226819));
#183137=CARTESIAN_POINT('Ctrl Pts',(77.5951651116529,-5.50056144135029,
76.2248244559558));
#183138=CARTESIAN_POINT('Ctrl Pts',(77.5820250984651,-5.5030758890797,76.2261868850227));
#183139=CARTESIAN_POINT('Ctrl Pts',(77.5690415015584,-5.5055023205584,76.2275226353722));
#183140=CARTESIAN_POINT('Ctrl Pts',(77.5625497031051,-5.50671553629776,
76.2281905105469));
#183141=CARTESIAN_POINT('Ctrl Pts',(77.5560970086979,-5.50790674721655,
76.2288517168236));
#183142=CARTESIAN_POINT('Ctrl Pts',(77.5496835246463,-5.50907638729464,
76.2295062352176));
#183143=CARTESIAN_POINT('Ctrl Pts',(77.5432700405948,-5.51024602737273,
76.2301607536115));
#183144=CARTESIAN_POINT('Ctrl Pts',(77.5413605897286,-5.51058776576927,
76.2303549106995));
#183145=CARTESIAN_POINT('Ctrl Pts',(77.5385278758308,-5.51110395017645,
76.2306491841668));
#183146=CARTESIAN_POINT('Ctrl Pts',(77.5225317368859,-5.51401880772868,
76.2323109260301));
#183147=CARTESIAN_POINT('Ctrl Pts',(77.502582434596,-5.51771225018848,76.2345019296031));
#183148=CARTESIAN_POINT('Ctrl Pts',(77.478663446348,-5.52205119172725,76.2372223822825));
#183149=CARTESIAN_POINT('Ctrl Pts',(77.4686964321468,-5.52385922355061,
76.2383559917064));
#183150=CARTESIAN_POINT('Ctrl Pts',(77.4580400637286,-5.52577871842334,
76.2395815452476));
#183151=CARTESIAN_POINT('Ctrl Pts',(77.4466929185927,-5.52779738571318,
76.2408990964935));
#183152=CARTESIAN_POINT('Ctrl Pts',(77.4194074079591,-5.53265150251016,
76.244067299429));
#183153=CARTESIAN_POINT('Ctrl Pts',(77.3881218669215,-5.53808546284043,
76.2477697163581));
#183154=CARTESIAN_POINT('Ctrl Pts',(77.3528552281582,-5.54401610952996,
76.252128643664));
#183155=CARTESIAN_POINT('Ctrl Pts',(77.3176159848871,-5.54994214923138,
76.2564841849097));
#183156=CARTESIAN_POINT('Ctrl Pts',(77.2784018478733,-5.55636409410674,
76.2614952132098));
#183157=CARTESIAN_POINT('Ctrl Pts',(77.2352213445396,-5.56314807052285,
76.2672855671192));
#183158=CARTESIAN_POINT('Ctrl Pts',(77.1994176836357,-5.56877309043764,
76.2720867123556));
#183159=CARTESIAN_POINT('Ctrl Pts',(77.1608868982291,-5.5746461130262,76.2774236884735));
#183160=CARTESIAN_POINT('Ctrl Pts',(77.1196285163624,-5.58066418896375,
76.2833680310246));
#183161=CARTESIAN_POINT('Ctrl Pts',(79.8067669157806,-4.75889434936128,
76.1478855624836));
#183162=CARTESIAN_POINT('Ctrl Pts',(79.4656552079978,-5.01633075955975,
76.2018288074578));
#183163=CARTESIAN_POINT('Ctrl Pts',(79.0981355517893,-5.2365440434876,76.2609701371046));
#183164=CARTESIAN_POINT('Ctrl Pts',(78.3757278221193,-5.56975423607527,
76.3785120140568));
#183165=CARTESIAN_POINT('Ctrl Pts',(78.0265892492644,-5.6926809850576,76.435791673461));
#183166=CARTESIAN_POINT('Ctrl Pts',(76.8543141967377,-5.98292457650376,
76.6272413549088));
#183167=CARTESIAN_POINT('Ctrl Pts',(76.0974424409179,-5.98222296632208,
76.7478529844076));
#183168=CARTESIAN_POINT('Ctrl Pts',(74.6929136633325,-5.77853241831115,
76.9740755107651));
#183169=CARTESIAN_POINT('Ctrl Pts',(73.9580143194339,-5.51877391939185,
77.0943934768112));
#183170=CARTESIAN_POINT('Ctrl Pts',(72.5747907323043,-4.69148727568362,
77.3177645343406));
#183171=CARTESIAN_POINT('Ctrl Pts',(72.0363102921168,-4.15598183372999,
77.4001313101903));
#183172=CARTESIAN_POINT('Ctrl Pts',(71.1810125590293,-3.02645959146061,
77.5298563962522));
#183173=CARTESIAN_POINT('Ctrl Pts',(70.83788218017,-2.32584157011803,77.5812538303274));
#183174=CARTESIAN_POINT('Ctrl Pts',(70.4329407787015,-0.802505729524864,
77.6328633583142));
#183175=CARTESIAN_POINT('Ctrl Pts',(70.4190230992651,-0.110255556371649,
77.6238715966117));
#183176=CARTESIAN_POINT('Ctrl Pts',(70.5275290426684,1.16543508448252,77.584711597924));
#183177=CARTESIAN_POINT('Ctrl Pts',(70.7286009034737,1.88783880921538,77.5393814133449));
#183178=CARTESIAN_POINT('Ctrl Pts',(71.3304192343141,3.10035853351918,77.4161289475591));
#183179=CARTESIAN_POINT('Ctrl Pts',(71.6869328784452,3.59894115111939,77.3445010729964));
#183180=CARTESIAN_POINT('Ctrl Pts',(72.5636028466731,4.48202484744894,77.1700775369511));
#183181=CARTESIAN_POINT('Ctrl Pts',(73.0815743965425,4.85387547286764,77.0691439922034));
#183182=CARTESIAN_POINT('Ctrl Pts',(74.0850504198822,5.34589610631609,76.8774557325446));
#183183=CARTESIAN_POINT('Ctrl Pts',(74.5994115705933,5.52772264370202,76.7805366540467));
#183184=CARTESIAN_POINT('Ctrl Pts',(75.1812918055743,5.62353578632127,76.6693002371056));
#183185=CARTESIAN_POINT('Origin',(76.1212924379081,7.14546725904962E-15,
76.2900208433682));
#183186=CARTESIAN_POINT('',(76.9592417890559,-4.82555798975984,76.1422677642937));
#183187=CARTESIAN_POINT('',(76.9592417890559,-4.82555798975984,76.1422677642937));
#183188=CARTESIAN_POINT('Origin',(76.1212924379081,7.14546725904962E-15,
76.2900208433682));
#183189=CARTESIAN_POINT('Origin',(76.0518331668413,7.15881389286582E-15,
75.8960977421633));
#183190=CARTESIAN_POINT('Ctrl Pts',(75.5161728246847,5.41644264198492,78.358216968557));
#183191=CARTESIAN_POINT('Ctrl Pts',(75.5019149418088,5.41387915560342,78.3610789631734));
#183192=CARTESIAN_POINT('Ctrl Pts',(75.4876667227446,5.41125711006823,78.3639371859045));
#183193=CARTESIAN_POINT('Ctrl Pts',(75.4255327841992,5.39955948906885,78.3763939104315));
#183194=CARTESIAN_POINT('Ctrl Pts',(75.3777553338061,5.38988133650626,78.3859530367993));
#183195=CARTESIAN_POINT('Ctrl Pts',(75.2023141057831,5.35181947554724,78.4209996640597));
#183196=CARTESIAN_POINT('Ctrl Pts',(75.0755278459142,5.31936972243571,78.4462199050885));
#183197=CARTESIAN_POINT('Ctrl Pts',(74.6674556431858,5.19871369377775,78.5273043409168));
#183198=CARTESIAN_POINT('Ctrl Pts',(74.3920524632714,5.09175193265122,78.5819143797841));
#183199=CARTESIAN_POINT('Ctrl Pts',(73.9919408034663,4.89679158174202,78.6620851728623));
#183200=CARTESIAN_POINT('Ctrl Pts',(73.8599693046185,4.82546805467803,78.6886699615825));
#183201=CARTESIAN_POINT('Ctrl Pts',(73.6629669240141,4.70803963466444,78.7286451726162));
#183202=CARTESIAN_POINT('Ctrl Pts',(73.5957227552475,4.66590460711774,78.7423440581148));
#183203=CARTESIAN_POINT('Ctrl Pts',(73.4687887813162,4.58238632244558,78.7683135508873));
#183204=CARTESIAN_POINT('Ctrl Pts',(73.4089578080457,4.54125565481166,78.780603409025));
#183205=CARTESIAN_POINT('Ctrl Pts',(73.2654826725282,4.43827687708175,78.8101969773947));
#183206=CARTESIAN_POINT('Ctrl Pts',(73.1827468240741,4.37517614643283,78.8273672647575));
#183207=CARTESIAN_POINT('Ctrl Pts',(73.0495032370545,4.26730323720836,78.8551891400921));
#183208=CARTESIAN_POINT('Ctrl Pts',(72.9979344986233,4.22392769921173,78.8660009081038));
#183209=CARTESIAN_POINT('Ctrl Pts',(72.7827710205176,4.03595398318632,78.9112892023277));
#183210=CARTESIAN_POINT('Ctrl Pts',(72.627068258779,3.8823362887325,78.9445183303616));
#183211=CARTESIAN_POINT('Ctrl Pts',(72.3674197499554,3.59322919644399,79.0004698999691));
#183212=CARTESIAN_POINT('Ctrl Pts',(72.2598282531279,3.4615325016442,79.0238463367233));
#183213=CARTESIAN_POINT('Ctrl Pts',(72.126388683757,3.28171624248632,79.0529321788238));
#183214=CARTESIAN_POINT('Ctrl Pts',(72.0949627144026,3.2380401493282,79.0597893570272));
#183215=CARTESIAN_POINT('Ctrl Pts',(72.0404809863824,3.15992587534142,79.0716818753935));
#183216=CARTESIAN_POINT('Ctrl Pts',(72.0171680308165,3.12568260712866,79.0767715519963));
#183217=CARTESIAN_POINT('Ctrl Pts',(71.9593347984207,3.03863717839425,79.089402433447));
#183218=CARTESIAN_POINT('Ctrl Pts',(71.9253246649039,2.9854892560426,79.0968358170441));
#183219=CARTESIAN_POINT('Ctrl Pts',(71.8500401207917,2.86326329726773,79.1133239695357));
#183220=CARTESIAN_POINT('Ctrl Pts',(71.8093429626874,2.79383145203852,79.1222618700749));
#183221=CARTESIAN_POINT('Ctrl Pts',(71.6654843506123,2.53559462668064,79.1540154782844));
#183222=CARTESIAN_POINT('Ctrl Pts',(71.5717832067193,2.34152844530379,79.1750271418635));
#183223=CARTESIAN_POINT('Ctrl Pts',(71.4159783056354,1.96386996730712,79.2111860569441));
#183224=CARTESIAN_POINT('Ctrl Pts',(71.3517094868113,1.78156216556626,79.2266902222285));
#183225=CARTESIAN_POINT('Ctrl Pts',(71.272853425363,1.51393382236065,79.2468650840652));
#183226=CARTESIAN_POINT('Ctrl Pts',(71.2505335000483,1.43114006228905,79.2527590812826));
#183227=CARTESIAN_POINT('Ctrl Pts',(71.212916840445,1.27749925141115,79.2630706292337));
#183228=CARTESIAN_POINT('Ctrl Pts',(71.197071431527,1.20681212166726,79.2675741632235));
#183229=CARTESIAN_POINT('Ctrl Pts',(71.1638143965143,1.04352771391044,79.2774301779147));
#183230=CARTESIAN_POINT('Ctrl Pts',(71.1473653971733,0.950748675231593,
79.282630338281));
#183231=CARTESIAN_POINT('Ctrl Pts',(71.0987046297217,0.628832684220777,
79.2992969798653));
#183232=CARTESIAN_POINT('Ctrl Pts',(71.0784338737235,0.398042190567016,
79.3088657223877));
#183233=CARTESIAN_POINT('Ctrl Pts',(71.0650214629203,-0.13113768080772,
79.3251419784573));
#183234=CARTESIAN_POINT('Ctrl Pts',(71.0813306320572,-0.429099154274402,
79.3302279709137));
#183235=CARTESIAN_POINT('Ctrl Pts',(71.1286500525202,-0.779286089998552,
79.3306584459885));
#183236=CARTESIAN_POINT('Ctrl Pts',(71.1368848392822,-0.834095414260751,
79.3305615796118));
#183237=CARTESIAN_POINT('Ctrl Pts',(71.1522371201957,-0.926906342177754,
79.3301095991703));
#183238=CARTESIAN_POINT('Ctrl Pts',(71.1589381318611,-0.964972346206565,
79.3298411076599));
#183239=CARTESIAN_POINT('Ctrl Pts',(71.1753298565719,-1.05277088847189,
79.3290287122979));
#183240=CARTESIAN_POINT('Ctrl Pts',(71.1853014783743,-1.1024457498079,79.3284261440093));
#183241=CARTESIAN_POINT('Ctrl Pts',(71.2261589107154,-1.29259243577014,
79.3255871590964));
#183242=CARTESIAN_POINT('Ctrl Pts',(71.2617679606139,-1.43197521063083,
79.3223860395607));
#183243=CARTESIAN_POINT('Ctrl Pts',(71.4090577741653,-1.92785125636295,
79.3072806067895));
#183244=CARTESIAN_POINT('Ctrl Pts',(71.5510006743666,-2.27410091233366,
79.2897519371849));
#183245=CARTESIAN_POINT('Ctrl Pts',(71.7754390299161,-2.69487242563776,
79.2606492921813));
#183246=CARTESIAN_POINT('Ctrl Pts',(71.826896158828,-2.78512661122168,79.2539029608224));
#183247=CARTESIAN_POINT('Ctrl Pts',(71.9189679329408,-2.93653286876974,
79.2417296143842));
#183248=CARTESIAN_POINT('Ctrl Pts',(71.9583209799575,-2.99843401826528,
79.2364978787745));
#183249=CARTESIAN_POINT('Ctrl Pts',(72.0434992184156,-3.12669664354118,
79.2251191556414));
#183250=CARTESIAN_POINT('Ctrl Pts',(72.0895680780906,-3.19287197127436,
79.2189343525147));
#183251=CARTESIAN_POINT('Ctrl Pts',(72.2304430038765,-3.38605207521559,
79.199933250951));
#183252=CARTESIAN_POINT('Ctrl Pts',(72.3292654508852,-3.50996138898529,
79.1864945487062));
#183253=CARTESIAN_POINT('Ctrl Pts',(72.6168449375001,-3.84023719191283,
79.1470199875352));
#183254=CARTESIAN_POINT('Ctrl Pts',(72.8161068343242,-4.03660894689595,
79.1192919068448));
#183255=CARTESIAN_POINT('Ctrl Pts',(73.1094564606271,-4.28461633682236,
79.0774156999498));
#183256=CARTESIAN_POINT('Ctrl Pts',(73.1916002571427,-4.3501070553025,79.0655847117028));
#183257=CARTESIAN_POINT('Ctrl Pts',(73.3137340347841,-4.44186336852166,
79.0477974946372));
#183258=CARTESIAN_POINT('Ctrl Pts',(73.3522957056441,-4.47005161992967,
79.0421540435315));
#183259=CARTESIAN_POINT('Ctrl Pts',(73.4271308736361,-4.52326632580226,
79.031143255864));
#183260=CARTESIAN_POINT('Ctrl Pts',(73.4633484032115,-4.5483667910836,79.0257881593876));
#183261=CARTESIAN_POINT('Ctrl Pts',(73.566677842625,-4.61814369924548,79.0104447268446));
#183262=CARTESIAN_POINT('Ctrl Pts',(73.6344655101185,-4.66176507802685,
79.0003025959736));
#183263=CARTESIAN_POINT('Ctrl Pts',(73.9024839516428,-4.82594167559996,
78.9599816255767));
#183264=CARTESIAN_POINT('Ctrl Pts',(74.1092700384102,-4.93495932705819,
78.9284116951794));
#183265=CARTESIAN_POINT('Ctrl Pts',(74.5219033964116,-5.11948179653936,
78.8652810353659));
#183266=CARTESIAN_POINT('Ctrl Pts',(74.7266043825922,-5.1964998340706,78.8339045344074));
#183267=CARTESIAN_POINT('Ctrl Pts',(75.0174649885859,-5.28619211479614,
78.7895055849814));
#183268=CARTESIAN_POINT('Ctrl Pts',(75.1001675666155,-5.3095446850927,78.7768999599303));
#183269=CARTESIAN_POINT('Ctrl Pts',(75.2528642273895,-5.34874328073306,
78.7536706468873));
#183270=CARTESIAN_POINT('Ctrl Pts',(75.3226869820234,-5.36518820000155,
78.7430656007244));
#183271=CARTESIAN_POINT('Ctrl Pts',(75.4828898687353,-5.39955722672238,
78.7187754382765));
#183272=CARTESIAN_POINT('Ctrl Pts',(75.5734412371254,-5.41656560554987,
78.705076482505));
#183273=CARTESIAN_POINT('Ctrl Pts',(75.7677510392994,-5.44792394359072,
78.6757449020032));
#183274=CARTESIAN_POINT('Ctrl Pts',(75.8715819611401,-5.46158604813196,
78.6601102245746));
#183275=CARTESIAN_POINT('Ctrl Pts',(76.1955068481785,-5.49462859427088,
78.6114320409621));
#183276=CARTESIAN_POINT('Ctrl Pts',(76.4164408094107,-5.50349609385866,
78.5783790890833));
#183277=CARTESIAN_POINT('Ctrl Pts',(76.8264814201847,-5.49471278816749,
78.5169938339591));
#183278=CARTESIAN_POINT('Ctrl Pts',(77.0153368711548,-5.48068641639614,
78.4887018730051));
#183279=CARTESIAN_POINT('Ctrl Pts',(77.2631393744103,-5.44907856650256,
78.4513197607304));
#183280=CARTESIAN_POINT('Ctrl Pts',(77.3230922441702,-5.44040040345994,
78.4422549071447));
#183281=CARTESIAN_POINT('Ctrl Pts',(77.4211723865814,-5.42450795093904,
78.4273798256251));
#183282=CARTESIAN_POINT('Ctrl Pts',(77.459391273806,-5.41789022187502,78.4215718442162));
#183283=CARTESIAN_POINT('Ctrl Pts',(77.5433125088904,-5.40242226517557,
78.4087904923963));
#183284=CARTESIAN_POINT('Ctrl Pts',(77.5889775534055,-5.39339114855114,
78.4018180259825));
#183285=CARTESIAN_POINT('Ctrl Pts',(77.7415687203998,-5.36115028822013,
78.3784729769647));
#183286=CARTESIAN_POINT('Ctrl Pts',(77.8479066865757,-5.33527112735,78.362127963739));
#183287=CARTESIAN_POINT('Ctrl Pts',(78.1430861425216,-5.25383017668497,
78.3166717234678));
#183288=CARTESIAN_POINT('Ctrl Pts',(78.3298148192446,-5.19112432475122,
78.2878219349732));
#183289=CARTESIAN_POINT('Ctrl Pts',(78.7276144333097,-5.03285944303159,
78.226638195943));
#183290=CARTESIAN_POINT('Ctrl Pts',(78.9368612656805,-4.9336454417792,78.1946390778234));
#183291=CARTESIAN_POINT('Ctrl Pts',(79.2233659394255,-4.77463192830892,
78.1514113034689));
#183292=CARTESIAN_POINT('Ctrl Pts',(79.3062001766343,-4.72574070304795,
78.138985175048));
#183293=CARTESIAN_POINT('Ctrl Pts',(79.4489054552507,-4.63633164728317,
78.1177189040025));
#183294=CARTESIAN_POINT('Ctrl Pts',(79.5093338267788,-4.59677817372079,
78.1087597913681));
#183295=CARTESIAN_POINT('Ctrl Pts',(79.6380270678341,-4.50884314507245,
78.0897833287989));
#183296=CARTESIAN_POINT('Ctrl Pts',(79.7060070644152,-4.46006503839995,
78.0798246067159));
#183297=CARTESIAN_POINT('Ctrl Pts',(79.9261175419339,-4.29434283709644,
78.0477958785182));
#183298=CARTESIAN_POINT('Ctrl Pts',(80.0733094384252,-4.17088753725781,
78.0267340503367));
#183299=CARTESIAN_POINT('Ctrl Pts',(80.4435224762492,-3.82569632497984,
77.9745685540693));
#183300=CARTESIAN_POINT('Ctrl Pts',(80.6546844161734,-3.59195896072616,
77.9456958990509));
#183301=CARTESIAN_POINT('Ctrl Pts',(80.8763084599508,-3.29977353857334,
77.9157044089384));
#183302=CARTESIAN_POINT('Ctrl Pts',(80.9071830097525,-3.2578466048847,77.9115334181342));
#183303=CARTESIAN_POINT('Ctrl Pts',(80.9618405150334,-3.18137248074178,
77.9041549939482));
#183304=CARTESIAN_POINT('Ctrl Pts',(80.9858308882512,-3.1469821006614,77.9009179604996));
#183305=CARTESIAN_POINT('Ctrl Pts',(81.0409034323538,-3.0660800580017,77.8934894978799));
#183306=CARTESIAN_POINT('Ctrl Pts',(81.0716756915484,-3.01936048596812,
77.889342011522));
#183307=CARTESIAN_POINT('Ctrl Pts',(81.1380644623453,-2.91514807754056,
77.8804152753713));
#183308=CARTESIAN_POINT('Ctrl Pts',(81.1733472509728,-2.85744933248507,
77.8756854361699));
#183309=CARTESIAN_POINT('Ctrl Pts',(81.282563414097,-2.67124958080769,77.8611250684101));
#183310=CARTESIAN_POINT('Ctrl Pts',(81.3524121887182,-2.5403807460344,77.8519394815153));
#183311=CARTESIAN_POINT('Ctrl Pts',(81.536092933521,-2.16031416155188,77.8284470977737));
#183312=CARTESIAN_POINT('Ctrl Pts',(81.6369084892845,-1.90518109225111,
77.8164300331646));
#183313=CARTESIAN_POINT('Ctrl Pts',(81.7459537131316,-1.55609387454003,
77.8053525438637));
#183314=CARTESIAN_POINT('Ctrl Pts',(81.771123771013,-1.46795901744542,77.8029916390186));
#183315=CARTESIAN_POINT('Ctrl Pts',(81.8122918970464,-1.30912810093927,
77.7995243082641));
#183316=CARTESIAN_POINT('Ctrl Pts',(81.8291022640084,-1.23866852137733,
77.7982588784447));
#183317=CARTESIAN_POINT('Ctrl Pts',(81.8633131017034,-1.08185818454473,
77.7960479721345));
#183318=CARTESIAN_POINT('Ctrl Pts',(81.8800532043596,-0.995382030637029,
77.7952308719302));
#183319=CARTESIAN_POINT('Ctrl Pts',(81.9330459170107,-0.682226280151792,
77.7937155384981));
#183320=CARTESIAN_POINT('Ctrl Pts',(81.9574005939911,-0.453763238979424,
77.7953287042204));
#183321=CARTESIAN_POINT('Ctrl Pts',(81.9815657321761,0.086629399831015,
77.8052474935193));
#183322=CARTESIAN_POINT('Ctrl Pts',(81.969468143672,0.398269146113887,77.8157320320428));
#183323=CARTESIAN_POINT('Ctrl Pts',(81.9242594577514,0.764723751114935,
77.8329103575786));
#183324=CARTESIAN_POINT('Ctrl Pts',(81.9162429635908,0.822257264086457,
77.8357499805543));
#183325=CARTESIAN_POINT('Ctrl Pts',(81.9013645814289,0.918001651934274,
77.8407042968495));
#183326=CARTESIAN_POINT('Ctrl Pts',(81.8950021199262,0.956288855472329,
77.8427465556726));
#183327=CARTESIAN_POINT('Ctrl Pts',(81.8797511257293,1.04245205493504,77.8474788586767));
#183328=CARTESIAN_POINT('Ctrl Pts',(81.8706330494829,1.09028123627393,77.8502020435365));
#183329=CARTESIAN_POINT('Ctrl Pts',(81.8476565059013,1.20272803807061,77.8568415540689));
#183330=CARTESIAN_POINT('Ctrl Pts',(81.8332705881775,1.26722546027236,77.86083586845));
#183331=CARTESIAN_POINT('Ctrl Pts',(81.7591987326617,1.57344650824585,77.8807376895099));
#183332=CARTESIAN_POINT('Ctrl Pts',(81.6844629328004,1.81106002175706,77.8989976824651));
#183333=CARTESIAN_POINT('Ctrl Pts',(81.5941173588847,2.04265365340619,77.9201017942693));
#183334=CARTESIAN_POINT('Ctrl Pts',(80.6284101054663,-3.63675684748496,
78.0903820385128));
#183335=CARTESIAN_POINT('Ctrl Pts',(80.3940563201404,-3.90523957448573,
78.1240877061337));
#183336=CARTESIAN_POINT('Ctrl Pts',(80.1345088331788,-4.14997445340766,
78.1625085719411));
#183337=CARTESIAN_POINT('Ctrl Pts',(79.7808318845804,-4.42352325093256,
78.214849052098));
#183338=CARTESIAN_POINT('Ctrl Pts',(79.70702012462,-4.47769516956664,78.2257760341449));
#183339=CARTESIAN_POINT('Ctrl Pts',(79.5728538380439,-4.57104850857269,
78.2456304732333));
#183340=CARTESIAN_POINT('Ctrl Pts',(79.5130143459865,-4.61094720078165,
78.254483335969));
#183341=CARTESIAN_POINT('Ctrl Pts',(79.3791100287484,-4.69644052719069,
78.2742841118123));
#183342=CARTESIAN_POINT('Ctrl Pts',(79.304711396019,-4.74146424476193,78.2852793300036));
#183343=CARTESIAN_POINT('Ctrl Pts',(79.0466088760025,-4.88930872787319,
78.3234016379376));
#183344=CARTESIAN_POINT('Ctrl Pts',(78.8580956201264,-4.98317373919724,
78.3512001122266));
#183345=CARTESIAN_POINT('Ctrl Pts',(78.4521140551989,-5.15662113600593,
78.4111396390857));
#183346=CARTESIAN_POINT('Ctrl Pts',(78.2340367450712,-5.23368833686723,
78.4433767616099));
#183347=CARTESIAN_POINT('Ctrl Pts',(77.8978367225211,-5.32877478829362,
78.4935205671464));
#183348=CARTESIAN_POINT('Ctrl Pts',(77.7828455378757,-5.35724758987058,
78.510749844654));
#183349=CARTESIAN_POINT('Ctrl Pts',(77.6204150291118,-5.39183777626021,
78.5352634496791));
#183350=CARTESIAN_POINT('Ctrl Pts',(77.5736585053054,-5.40114850324744,
78.5423401715031));
#183351=CARTESIAN_POINT('Ctrl Pts',(77.4888987347911,-5.41686141270102,
78.5552117338151));
#183352=CARTESIAN_POINT('Ctrl Pts',(77.4509374536727,-5.42347852051812,
78.5609926054656));
#183353=CARTESIAN_POINT('Ctrl Pts',(77.3552234922236,-5.43910673546241,
78.5756056383617));
#183354=CARTESIAN_POINT('Ctrl Pts',(77.2973938582507,-5.44758530027873,
78.5844681789869));
#183355=CARTESIAN_POINT('Ctrl Pts',(76.9408425364603,-5.49394270818737,
78.6392701766296));
#183356=CARTESIAN_POINT('Ctrl Pts',(76.6396746582074,-5.50761552944876,
78.6862191406364));
#183357=CARTESIAN_POINT('Ctrl Pts',(76.1081481615792,-5.48707644632523,
78.7687619288734));
#183358=CARTESIAN_POINT('Ctrl Pts',(75.8781766930943,-5.46329221801716,
78.8043742861795));
#183359=CARTESIAN_POINT('Ctrl Pts',(75.5642555778109,-5.41023515989713,
78.8525584951231));
#183360=CARTESIAN_POINT('Ctrl Pts',(75.4785158118147,-5.39358996277604,
78.8656756805764));
#183361=CARTESIAN_POINT('Ctrl Pts',(75.3232229171448,-5.35950561308275,
78.8893455537025));
#183362=CARTESIAN_POINT('Ctrl Pts',(75.2535458744884,-5.34275035193755,
78.8999331124092));
#183363=CARTESIAN_POINT('Ctrl Pts',(75.0967208734763,-5.30171714388795,
78.9236863785074));
#183364=CARTESIAN_POINT('Ctrl Pts',(75.0098001927731,-5.27662465662882,
78.9367973825715));
#183365=CARTESIAN_POINT('Ctrl Pts',(74.6573841534686,-5.16522700102426,
78.9897383307418));
#183366=CARTESIAN_POINT('Ctrl Pts',(74.3979441995,-5.06054142428486,79.0281768308309));
#183367=CARTESIAN_POINT('Ctrl Pts',(73.9624528718956,-4.84432950924887,
79.0922309979064));
#183368=CARTESIAN_POINT('Ctrl Pts',(73.7826456927854,-4.74187732155216,
79.1185340890117));
#183369=CARTESIAN_POINT('Ctrl Pts',(73.5619592860798,-4.59885388815738,
79.1509129254303));
#183370=CARTESIAN_POINT('Ctrl Pts',(73.5153486181535,-4.5676108729711,79.1577577753707));
#183371=CARTESIAN_POINT('Ctrl Pts',(73.4349332402378,-4.51188419364041,
79.1695871865049));
#183372=CARTESIAN_POINT('Ctrl Pts',(73.4009149150978,-4.48772543288065,
79.1745986299192));
#183373=CARTESIAN_POINT('Ctrl Pts',(73.3255623119591,-4.43289659231789,
79.1857137727034));
#183374=CARTESIAN_POINT('Ctrl Pts',(73.2843775456728,-4.40202593011779,
79.1917980324538));
#183375=CARTESIAN_POINT('Ctrl Pts',(73.0278240876535,-4.20397924862833,
79.2297260779207));
#183376=CARTESIAN_POINT('Ctrl Pts',(72.8246717576473,-4.02129618245288,
79.2598638888135));
#183377=CARTESIAN_POINT('Ctrl Pts',(72.5288581331804,-3.71241269160276,
79.3029618475044));
#183378=CARTESIAN_POINT('Ctrl Pts',(72.4266454204006,-3.59625080900249,
79.317684432372));
#183379=CARTESIAN_POINT('Ctrl Pts',(72.2944934548233,-3.43267559169422,
79.336379003805));
#183380=CARTESIAN_POINT('Ctrl Pts',(72.2602379570709,-3.38894090182474,
79.3411912480854));
#183381=CARTESIAN_POINT('Ctrl Pts',(72.1709185412686,-3.27129332051794,
79.3536413916588));
#183382=CARTESIAN_POINT('Ctrl Pts',(72.1170219598297,-3.19649294736063,
79.3610508654127));
#183383=CARTESIAN_POINT('Ctrl Pts',(72.0242364371869,-3.06069810282558,
79.3736026796211));
#183384=CARTESIAN_POINT('Ctrl Pts',(71.984632835931,-3.00023200104705,79.3788874996497));
#183385=CARTESIAN_POINT('Ctrl Pts',(71.8998700738488,-2.86513080676946,
79.3900292429983));
#183386=CARTESIAN_POINT('Ctrl Pts',(71.855261605413,-2.79016461705903,79.3957777141826));
#183387=CARTESIAN_POINT('Ctrl Pts',(71.7199375449584,-2.55006098473281,
79.4128375044416));
#183388=CARTESIAN_POINT('Ctrl Pts',(71.635799810449,-2.38128295559807,79.4228577158204));
#183389=CARTESIAN_POINT('Ctrl Pts',(71.4596352730075,-1.9778330699217,79.4424495112208));
#183390=CARTESIAN_POINT('Ctrl Pts',(71.3746112017346,-1.74049959752493,
79.4507174097963));
#183391=CARTESIAN_POINT('Ctrl Pts',(71.2721440191207,-1.37894573163261,
79.4590399499996));
#183392=CARTESIAN_POINT('Ctrl Pts',(71.2423410997523,-1.25861494621162,
79.4611340684039));
#183393=CARTESIAN_POINT('Ctrl Pts',(71.2064670197567,-1.08976108210987,
79.4632119915069));
#183394=CARTESIAN_POINT('Ctrl Pts',(71.1969755268986,-1.04200825367281,
79.4637051033297));
#183395=CARTESIAN_POINT('Ctrl Pts',(71.1810361070769,-0.955908735576465,
79.4644308674772));
#183396=CARTESIAN_POINT('Ctrl Pts',(71.1743609744854,-0.917608665010389,
79.4646965431651));
#183397=CARTESIAN_POINT('Ctrl Pts',(71.1586852474065,-0.821725018920534,
79.4652164002841));
#183398=CARTESIAN_POINT('Ctrl Pts',(71.1501877132287,-0.764064033727843,
79.4653979356255));
#183399=CARTESIAN_POINT('Ctrl Pts',(71.1076577202557,-0.440270866784525,
79.4656456398651));
#183400=CARTESIAN_POINT('Ctrl Pts',(71.0920073221885,-0.172091960468779,
79.4629227734747));
#183401=CARTESIAN_POINT('Ctrl Pts',(71.0991580243968,0.350936268173423,
79.4508351450115));
#183402=CARTESIAN_POINT('Ctrl Pts',(71.1200712756766,0.605142448434162,
79.4418208995794));
#183403=CARTESIAN_POINT('Ctrl Pts',(71.1723404022888,0.950155925792415,
79.4248786898478));
#183404=CARTESIAN_POINT('Ctrl Pts',(71.1888257930237,1.04302556978188,79.4198443371493));
#183405=CARTESIAN_POINT('Ctrl Pts',(71.2221157607872,1.20640586945421,79.4101341632058));
#183406=CARTESIAN_POINT('Ctrl Pts',(71.2379598424545,1.27709975656437,79.4056461538721));
#183407=CARTESIAN_POINT('Ctrl Pts',(71.275538324518,1.43068751965561,79.3952648021893));
#183408=CARTESIAN_POINT('Ctrl Pts',(71.2978148466917,1.51342192875155,79.3892660070318));
#183409=CARTESIAN_POINT('Ctrl Pts',(71.3755412456854,1.7776551228409,79.3687943117415));
#183410=CARTESIAN_POINT('Ctrl Pts',(71.4383370514556,1.95673625253443,79.3528961839455));
#183411=CARTESIAN_POINT('Ctrl Pts',(71.5927942206316,2.33404340058379,79.3151060344769));
#183412=CARTESIAN_POINT('Ctrl Pts',(71.687250033547,2.53072517927569,79.2927029141657));
#183413=CARTESIAN_POINT('Ctrl Pts',(71.8323248734623,2.79183004607981,79.2594347535072));
#183414=CARTESIAN_POINT('Ctrl Pts',(71.873168083406,2.86165644053519,79.25017236789));
#183415=CARTESIAN_POINT('Ctrl Pts',(71.9487109790548,2.9844787968286,79.2332448050653));
#183416=CARTESIAN_POINT('Ctrl Pts',(71.9828186985332,3.03783417992675,79.2256697004847));
#183417=CARTESIAN_POINT('Ctrl Pts',(72.0407671796245,3.1251013311687,79.2129215174997));
#183418=CARTESIAN_POINT('Ctrl Pts',(72.0640851696806,3.15936321495012,79.2078229453833));
#183419=CARTESIAN_POINT('Ctrl Pts',(72.1184875630804,3.23737116557289,79.195999609947));
#183420=CARTESIAN_POINT('Ctrl Pts',(72.1498286991465,3.28092604623859,79.1892387131608));
#183421=CARTESIAN_POINT('Ctrl Pts',(72.2889760397257,3.46839919845321,79.1594124026569));
#183422=CARTESIAN_POINT('Ctrl Pts',(72.4031530541565,3.60729666314041,79.1354176121167));
#183423=CARTESIAN_POINT('Ctrl Pts',(72.6669339258392,3.89764530905349,79.0805469864712));
#183424=CARTESIAN_POINT('Ctrl Pts',(72.818955314213,4.04641685705457,79.0492630652738));
#183425=CARTESIAN_POINT('Ctrl Pts',(73.0552477582408,4.25194759286441,79.0007659498778));
#183426=CARTESIAN_POINT('Ctrl Pts',(73.1331654950865,4.31598509597362,78.9847941829096));
#183427=CARTESIAN_POINT('Ctrl Pts',(73.283061693228,4.43231073131682,78.9540751337371));
#183428=CARTESIAN_POINT('Ctrl Pts',(73.3546414089213,4.48507802032732,78.9394088384307));
#183429=CARTESIAN_POINT('Ctrl Pts',(73.4859728498022,4.57696959325129,78.9124922524133));
#183430=CARTESIAN_POINT('Ctrl Pts',(73.545273544558,4.61672886589895,78.9003359173442));
#183431=CARTESIAN_POINT('Ctrl Pts',(73.6795295275472,4.70292096621732,78.8728043387005));
#183432=CARTESIAN_POINT('Ctrl Pts',(73.7548601082599,4.74870513158792,78.8573497454659));
#183433=CARTESIAN_POINT('Ctrl Pts',(74.0288519637286,4.90612330707909,78.8011143468831));
#183434=CARTESIAN_POINT('Ctrl Pts',(74.2332640466902,5.00681107205553,78.7591039745079));
#183435=CARTESIAN_POINT('Ctrl Pts',(74.6382203141554,5.17503856381936,78.6759928941913));
#183436=CARTESIAN_POINT('Ctrl Pts',(74.8376431273674,5.24429695495903,78.6351170892154));
#183437=CARTESIAN_POINT('Ctrl Pts',(75.1492114923075,5.33209345712713,78.5716548166039));
#183438=CARTESIAN_POINT('Ctrl Pts',(75.2587846491163,5.35922531673406,78.5494115242861));
#183439=CARTESIAN_POINT('Ctrl Pts',(75.4148252560965,5.39260979731577,78.517902015241));
#183440=CARTESIAN_POINT('Ctrl Pts',(75.4606446248287,5.4017802055123,78.5086697873934));
#183441=CARTESIAN_POINT('Ctrl Pts',(75.5176778258127,5.41241160737266,78.4972071924153));
#183442=CARTESIAN_POINT('Ctrl Pts',(75.5287827382832,5.41444490413952,78.4949766817791));
#183443=CARTESIAN_POINT('Ctrl Pts',(75.539893974202,5.41644264127421,78.4927463157663));
#183444=CARTESIAN_POINT('Origin',(81.0480631074551,0.,102.742429499351));
#183445=CARTESIAN_POINT('',(68.2357429722793,-7.92639144670273E-16,67.3531585631293));
#183446=CARTESIAN_POINT('Origin',(74.6098026240559,0.,66.2292398698762));
#183447=CARTESIAN_POINT('',(68.1557866073341,-7.92639144670273E-16,66.8997034842526));
#183448=CARTESIAN_POINT('',(74.6740034556784,-7.92639144670273E-16,103.866348192604));
#183449=CARTESIAN_POINT('Origin',(74.5298462591107,0.,65.7757847909995));
#183450=CARTESIAN_POINT('Origin',(74.404241366658,0.,65.0634440479771));
#183451=CARTESIAN_POINT('',(67.9045768224286,-7.9263914467027E-16,65.4750219982078));
#183452=CARTESIAN_POINT('Origin',(68.6509091160486,-7.15449274600975E-16,
66.0779117527394));
#183453=CARTESIAN_POINT('Origin',(74.2786364742053,0.,64.3511033049547));
#183454=CARTESIAN_POINT('Origin',(81.0480631074551,0.,102.742429499351));
#183455=CARTESIAN_POINT('',(67.8248987953766,-7.92639144670271E-16,65.0231454519647));
#183456=CARTESIAN_POINT('',(74.6740034556784,-7.92639144670271E-16,103.866348192604));
#183457=CARTESIAN_POINT('Origin',(74.1989584471533,0.,63.8992267587115));
#183458=CARTESIAN_POINT('Origin',(78.1406475300671,0.,87.742352664884));
#183459=CARTESIAN_POINT('',(90.3032326828481,1.10218211923262E-15,104.890866373114));
#183460=CARTESIAN_POINT('',(72.5766931286283,-1.10218211923262E-15,108.016533571118));
#183461=CARTESIAN_POINT('Origin',(81.4399629057382,0.,106.453699972116));
#183462=CARTESIAN_POINT('',(69.2773777529572,-1.10218211923262E-15,89.3051862638862));
#183463=CARTESIAN_POINT('',(69.2773777529572,-1.10218211923262E-15,89.3051862638862));
#183464=CARTESIAN_POINT('Origin',(78.1406475300671,0.,87.742352664884));
#183465=CARTESIAN_POINT('Origin',(81.4399629057382,0.,106.453699972116));
#183466=CARTESIAN_POINT('Origin',(81.5267869945717,5.42101086242752E-17,
106.946103848622));
#183467=CARTESIAN_POINT('',(71.9391817309499,-1.17043669052308E-15,110.159797254809));
#183468=CARTESIAN_POINT('Origin',(81.787259261072,5.42101086242752E-17,
108.42331547814));
#183469=CARTESIAN_POINT('',(71.765533553283,-1.17043669052308E-15,109.174989501797));
#183470=CARTESIAN_POINT('',(71.6787094644496,-1.17043669052308E-15,108.682585625291));
#183471=CARTESIAN_POINT('',(91.4616886135273,1.27885690777163E-15,105.702025948459));
#183472=CARTESIAN_POINT('Origin',(81.6136110834051,5.42101086242752E-17,
107.438507725128));
#183473=CARTESIAN_POINT('Origin',(81.6136110834051,5.42101086242752E-17,
107.438507725128));
#183474=CARTESIAN_POINT('Origin',(81.787259261072,5.42101086242752E-17,
108.42331547814));
#183475=CARTESIAN_POINT('',(72.5184096962895,-1.10920435056572E-15,110.565377042483));
#183476=CARTESIAN_POINT('Origin',(81.8740833499055,5.42101086242752E-17,
108.915719354647));
#183477=CARTESIAN_POINT('Origin',(72.431585607456,-1.10920435056571E-15,
110.072973165976));
#183478=CARTESIAN_POINT('Origin',(81.6136110834051,5.42101086242752E-17,
107.438507725128));
#183479=CARTESIAN_POINT('',(90.8824606481877,-1.10920435056571E-15,105.296446160786));
#183480=CARTESIAN_POINT('Origin',(81.5267869945717,5.42101086242752E-17,
106.946103848622));
#183481=CARTESIAN_POINT('Origin',(90.9692847370211,-1.10920435056571E-15,
105.788850037292));
#183482=CARTESIAN_POINT('Origin',(81.4399629057382,0.,106.453699972116));
#183483=CARTESIAN_POINT('Origin',(90.7956365593542,-1.16341445918999E-15,
104.80404228428));
#183484=CARTESIAN_POINT('Origin',(78.1406475300671,0.,87.742352664884));
#183485=CARTESIAN_POINT('',(70.2621855059694,-9.79717439317882E-16,89.1315380862193));
#183486=CARTESIAN_POINT('Origin',(78.1406475300671,0.,87.742352664884));
#183487=CARTESIAN_POINT('',(73.5615008816405,-9.79717439317882E-16,107.842885393451));
#183488=CARTESIAN_POINT('',(70.2621855059694,-9.79717439317882E-16,89.1315380862193));
#183489=CARTESIAN_POINT('Origin',(81.4399629057382,0.,106.453699972116));
#183490=CARTESIAN_POINT('Origin',(81.4399629057382,0.,106.453699972116));
#183491=CARTESIAN_POINT('',(74.1407288469801,-9.18485099360508E-16,108.248465181124));
#183492=CARTESIAN_POINT('Origin',(74.0539047581466,-9.18485099360515E-16,
107.756061304618));
#183493=CARTESIAN_POINT('Origin',(81.5267869945717,0.,106.946103848622));
#183494=CARTESIAN_POINT('Origin',(81.5267869945717,0.,106.946103848622));
#183495=CARTESIAN_POINT('',(84.4241289406192,-4.89858719658941E-16,100.342664619881));
#183496=CARTESIAN_POINT('Origin',(80.4848979285703,0.,101.037257330549));
#183497=CARTESIAN_POINT('',(85.4660180066205,-4.89858719658941E-16,106.251511137954));
#183498=CARTESIAN_POINT('',(85.4660180066205,-4.89858719658941E-16,106.251511137954));
#183499=CARTESIAN_POINT('Origin',(81.5267869945717,0.,106.946103848622));
#183500=CARTESIAN_POINT('Origin',(81.0480631074551,0.,102.742429499351));
#183501=CARTESIAN_POINT('',(78.4660420348953,-2.827108640986E-16,101.393236094766));
#183502=CARTESIAN_POINT('Origin',(80.7394799846693,0.,100.992367645255));
#183503=CARTESIAN_POINT('',(72.336364674282,-2.827108640986E-16,66.6301083193878));
#183504=CARTESIAN_POINT('',(78.7746251576811,-2.827108640986E-16,103.143297948862));
#183505=CARTESIAN_POINT('Origin',(74.609802624056,0.,66.2292398698762));
#183506=CARTESIAN_POINT('Origin',(80.4848979285703,0.,101.037257330549));
#183507=CARTESIAN_POINT('Origin',(81.5267869945717,0.,106.946103848622));
#183508=CARTESIAN_POINT('Origin',(81.8740833499055,5.42101086242752E-17,
108.915719354647));
#183509=CARTESIAN_POINT('Origin',(78.1406475300671,0.,87.742352664884));
#183510=CARTESIAN_POINT('Origin',(74.1989584471533,0.,63.8992267587115));
#183511=CARTESIAN_POINT('Origin',(80.9838622758326,0.,65.1053211766231));
#183512=CARTESIAN_POINT('Ctrl Pts',(75.1292776351945,5.33099171449205,76.0772561825838));
#183513=CARTESIAN_POINT('Ctrl Pts',(73.7606186056544,5.08490089911617,76.3524352506115));
#183514=CARTESIAN_POINT('Ctrl Pts',(71.234833133868,3.43952652893016,76.8654944842279));
#183515=CARTESIAN_POINT('Ctrl Pts',(70.2709209865568,-1.04183990292265,
77.13700086402));
#183516=CARTESIAN_POINT('Ctrl Pts',(72.7198166924919,-4.91215295642792,
76.8067371393112));
#183517=CARTESIAN_POINT('Ctrl Pts',(77.1504659164359,-5.90856770039853,
76.1270368002636));
#183518=CARTESIAN_POINT('Ctrl Pts',(80.9793450358789,-3.43952652893015,
75.5534447668232));
#183519=CARTESIAN_POINT('Ctrl Pts',(81.9779868187236,1.04183990292267,75.4788999376335));
#183520=CARTESIAN_POINT('Ctrl Pts',(79.5638207483218,4.91215295642794,76.0061252129447));
#183521=CARTESIAN_POINT('Ctrl Pts',(75.1679011599112,5.90856770039855,76.8827871025948));
#183522=CARTESIAN_POINT('Ctrl Pts',(71.3737516760015,3.43952652893017,77.6533406866376));
#183523=CARTESIAN_POINT('Ctrl Pts',(70.4098395286903,-1.04183990292265,
77.9248470664298));
#183524=CARTESIAN_POINT('Ctrl Pts',(72.8587352346254,-4.91215295642792,
77.594583341721));
#183525=CARTESIAN_POINT('Ctrl Pts',(77.2893844585694,-5.90856770039853,
76.9148830026733));
#183526=CARTESIAN_POINT('Ctrl Pts',(81.1182635780125,-3.43952652893014,
76.3412909692329));
#183527=CARTESIAN_POINT('Ctrl Pts',(82.1169053608571,1.04183990292266,76.2667461400432));
#183528=CARTESIAN_POINT('Ctrl Pts',(79.7027392904554,4.91215295642793,76.7939714153545));
#183529=CARTESIAN_POINT('Ctrl Pts',(75.3068197020447,5.90856770039855,77.6706333050046));
#183530=CARTESIAN_POINT('Ctrl Pts',(71.512670218135,3.43952652893016,78.4411868890474));
#183531=CARTESIAN_POINT('Ctrl Pts',(70.5487580708238,-1.04183990292265,
78.7126932688396));
#183532=CARTESIAN_POINT('Ctrl Pts',(72.9976537767589,-4.91215295642791,
78.3824295441307));
#183533=CARTESIAN_POINT('Ctrl Pts',(77.4283030007029,-5.90856770039854,
77.7027292050831));
#183534=CARTESIAN_POINT('Ctrl Pts',(81.257182120146,-3.43952652893014,77.1291371716427));
#183535=CARTESIAN_POINT('Ctrl Pts',(82.2558239029906,1.04183990292265,77.054592342453));
#183536=CARTESIAN_POINT('Ctrl Pts',(79.8416578325889,4.91215295642793,77.5818176177643));
#183537=CARTESIAN_POINT('Ctrl Pts',(75.4457382441782,5.90856770039855,78.4584795074144));
#183538=CARTESIAN_POINT('Ctrl Pts',(71.6515887602686,3.43952652893016,79.2290330914572));
#183539=CARTESIAN_POINT('Ctrl Pts',(70.6876766129573,-1.04183990292266,
79.5005394712493));
#183540=CARTESIAN_POINT('Ctrl Pts',(73.1365723188924,-4.91215295642791,
79.1702757465405));
#183541=CARTESIAN_POINT('Ctrl Pts',(77.5672215428365,-5.90856770039854,
78.4905754074929));
#183542=CARTESIAN_POINT('Ctrl Pts',(81.3961006622795,-3.43952652893014,
77.9169833740525));
#183543=CARTESIAN_POINT('Ctrl Pts',(82.3947424451241,1.04183990292264,77.8424385448628));
#183544=CARTESIAN_POINT('Ctrl Pts',(79.9805763747224,4.91215295642793,78.369663820174));
#183545=CARTESIAN_POINT('Ctrl Pts',(75.5846567863118,5.90856770039855,79.2463257098241));
#183546=CARTESIAN_POINT('Ctrl Pts',(71.7905073024021,3.43952652893017,80.016879293867));
#183547=CARTESIAN_POINT('Ctrl Pts',(70.8265951550908,-1.04183990292266,
80.2883856736591));
#183548=CARTESIAN_POINT('Ctrl Pts',(73.2754908610259,-4.91215295642791,
79.9581219489503));
#183549=CARTESIAN_POINT('Ctrl Pts',(77.70614008497,-5.90856770039854,79.2784216099027));
#183550=CARTESIAN_POINT('Ctrl Pts',(81.535019204413,-3.43952652893014,78.7048295764623));
#183551=CARTESIAN_POINT('Ctrl Pts',(82.5336609872576,1.04183990292264,78.6302847472725));
#183552=CARTESIAN_POINT('Ctrl Pts',(80.1194949168559,4.91215295642793,79.1575100225838));
#183553=CARTESIAN_POINT('Ctrl Pts',(75.7235753284453,5.90856770039854,80.0341719122339));
#183554=CARTESIAN_POINT('Ctrl Pts',(71.9294258445356,3.4395265289302,80.8047254962767));
#183555=CARTESIAN_POINT('Ctrl Pts',(70.9655136972244,-1.04183990292267,
81.0762318760689));
#183556=CARTESIAN_POINT('Ctrl Pts',(73.4144094031595,-4.91215295642791,
80.7459681513601));
#183557=CARTESIAN_POINT('Ctrl Pts',(77.8450586271034,-5.90856770039855,
80.0662678123124));
#183558=CARTESIAN_POINT('Ctrl Pts',(81.6739377465466,-3.43952652893014,
79.492675778872));
#183559=CARTESIAN_POINT('Ctrl Pts',(82.6725795293912,1.04183990292264,79.4181309496823));
#183560=CARTESIAN_POINT('Ctrl Pts',(80.2584134589894,4.91215295642795,79.9453562249936));
#183561=CARTESIAN_POINT('Ctrl Pts',(75.8624938705788,5.90856770039853,80.8220181146437));
#183562=CARTESIAN_POINT('Ctrl Pts',(72.0683443866692,3.4395265289302,81.5925716986865));
#183563=CARTESIAN_POINT('Ctrl Pts',(71.294008903086,-0.160470683265631,
81.810679774696));
#183564=CARTESIAN_POINT('Ctrl Pts',(71.9717750339029,-2.06421305036014,
81.738895603627));
#183565=CARTESIAN_POINT('Ctrl Pts',(72.248017627255,-2.57465544021205,81.704063311873));
#183566=CARTESIAN_POINT('Ctrl Pts',(75.0835432977388,5.96755461207746,76.4642667723862));
#183567=CARTESIAN_POINT('Ctrl Pts',(73.5507643062705,5.69207859205401,76.7683846177746));
#183568=CARTESIAN_POINT('Ctrl Pts',(70.7219975874206,3.8502334087825,77.334867619897));
#183569=CARTESIAN_POINT('Ctrl Pts',(69.6409131499095,-1.16624389057502,
77.6270346358428));
#183570=CARTESIAN_POINT('Ctrl Pts',(72.3801530226782,-5.49870316824427,
77.2455754008299));
#183571=CARTESIAN_POINT('Ctrl Pts',(77.3377835776619,-6.61409777385948,
76.4729540347903));
#183572=CARTESIAN_POINT('Ctrl Pts',(81.621787881687,-3.85023340878249,75.8191111517082));
#183573=CARTESIAN_POINT('Ctrl Pts',(82.7376019547315,1.16624389057504,75.7239056863648));
#183574=CARTESIAN_POINT('Ctrl Pts',(80.0330917174962,5.49870316824429,76.3023264719802));
#183575=CARTESIAN_POINT('Ctrl Pts',(75.1101907980458,6.61409777385949,77.2719093886222));
#183576=CARTESIAN_POINT('Ctrl Pts',(70.8609161295542,3.8502334087825,78.1227138223068));
#183577=CARTESIAN_POINT('Ctrl Pts',(69.779831692043,-1.16624389057502,78.4148808382526));
#183578=CARTESIAN_POINT('Ctrl Pts',(72.5190715648117,-5.49870316824427,
78.0334216032397));
#183579=CARTESIAN_POINT('Ctrl Pts',(77.4767021197954,-6.61409777385948,
77.2608002372001));
#183580=CARTESIAN_POINT('Ctrl Pts',(81.7607064238205,-3.85023340878248,
76.606957354118));
#183581=CARTESIAN_POINT('Ctrl Pts',(82.876520496865,1.16624389057503,76.5117518887746));
#183582=CARTESIAN_POINT('Ctrl Pts',(80.1720102596297,5.49870316824428,77.0901726743899));
#183583=CARTESIAN_POINT('Ctrl Pts',(75.2491093401794,6.6140977738595,78.059755591032));
#183584=CARTESIAN_POINT('Ctrl Pts',(70.9998346716877,3.85023340878249,78.9105600247165));
#183585=CARTESIAN_POINT('Ctrl Pts',(69.9187502341765,-1.16624389057502,
79.2027270406623));
#183586=CARTESIAN_POINT('Ctrl Pts',(72.6579901069452,-5.49870316824426,
78.8212678056494));
#183587=CARTESIAN_POINT('Ctrl Pts',(77.615620661929,-6.61409777385948,78.0486464396098));
#183588=CARTESIAN_POINT('Ctrl Pts',(81.899624965954,-3.85023340878247,77.3948035565277));
#183589=CARTESIAN_POINT('Ctrl Pts',(83.0154390389986,1.16624389057501,77.2995980911844));
#183590=CARTESIAN_POINT('Ctrl Pts',(80.3109288017633,5.49870316824428,77.8780188767997));
#183591=CARTESIAN_POINT('Ctrl Pts',(75.3880278823129,6.61409777385949,78.8476017934417));
#183592=CARTESIAN_POINT('Ctrl Pts',(71.1387532138212,3.8502334087825,79.6984062271263));
#183593=CARTESIAN_POINT('Ctrl Pts',(70.0576687763101,-1.16624389057503,
79.9905732430721));
#183594=CARTESIAN_POINT('Ctrl Pts',(72.7969086490787,-5.49870316824426,
79.6091140080592));
#183595=CARTESIAN_POINT('Ctrl Pts',(77.7545392040625,-6.61409777385948,
78.8364926420196));
#183596=CARTESIAN_POINT('Ctrl Pts',(82.0385435080876,-3.85023340878247,
78.1826497589375));
#183597=CARTESIAN_POINT('Ctrl Pts',(83.1543575811321,1.16624389057501,78.0874442935942));
#183598=CARTESIAN_POINT('Ctrl Pts',(80.4498473438968,5.49870316824428,78.6658650792095));
#183599=CARTESIAN_POINT('Ctrl Pts',(75.5269464244464,6.61409777385949,79.6354479958515));
#183600=CARTESIAN_POINT('Ctrl Pts',(71.2776717559547,3.8502334087825,80.4862524295361));
#183601=CARTESIAN_POINT('Ctrl Pts',(70.1965873184436,-1.16624389057503,
80.7784194454819));
#183602=CARTESIAN_POINT('Ctrl Pts',(72.9358271912123,-5.49870316824426,
80.396960210469));
#183603=CARTESIAN_POINT('Ctrl Pts',(77.893457746196,-6.61409777385948,79.6243388444294));
#183604=CARTESIAN_POINT('Ctrl Pts',(82.1774620502211,-3.85023340878248,
78.9704959613473));
#183605=CARTESIAN_POINT('Ctrl Pts',(83.2932761232656,1.16624389057501,78.8752904960039));
#183606=CARTESIAN_POINT('Ctrl Pts',(80.5887658860303,5.49870316824428,79.4537112816192));
#183607=CARTESIAN_POINT('Ctrl Pts',(75.6658649665799,6.61409777385948,80.4232941982613));
#183608=CARTESIAN_POINT('Ctrl Pts',(71.4165902980883,3.85023340878254,81.2740986319458));
#183609=CARTESIAN_POINT('Ctrl Pts',(70.3355058605771,-1.16624389057504,
81.5662656478916));
#183610=CARTESIAN_POINT('Ctrl Pts',(73.0747457333458,-5.49870316824426,
81.1848064128787));
#183611=CARTESIAN_POINT('Ctrl Pts',(78.0323762883295,-6.61409777385949,
80.4121850468392));
#183612=CARTESIAN_POINT('Ctrl Pts',(82.3163805923546,-3.85023340878247,
79.7583421637571));
#183613=CARTESIAN_POINT('Ctrl Pts',(83.4321946653991,1.166243890575,79.6631366984137));
#183614=CARTESIAN_POINT('Ctrl Pts',(80.7276844281638,5.49870316824431,80.241557484029));
#183615=CARTESIAN_POINT('Ctrl Pts',(75.8047835087135,6.61409777385948,81.2111404006711));
#183616=CARTESIAN_POINT('Ctrl Pts',(71.5555088402218,3.85023340878254,82.0619448343556));
#183617=CARTESIAN_POINT('Ctrl Pts',(70.6870458344909,-0.179632161764912,
82.296650132147));
#183618=CARTESIAN_POINT('Ctrl Pts',(71.4447681147403,-2.31069653991403,
82.2107675346595));
#183619=CARTESIAN_POINT('Ctrl Pts',(71.7537129129724,-2.88208981923202,
82.1701689618565));
#183620=CARTESIAN_POINT('Ctrl Pts',(74.9476130689139,5.96755461207746,75.6933681369149));
#183621=CARTESIAN_POINT('Ctrl Pts',(73.4148340774456,5.69207859205401,75.9974859823033));
#183622=CARTESIAN_POINT('Ctrl Pts',(70.5860673585957,3.8502334087825,76.5639689844257));
#183623=CARTESIAN_POINT('Ctrl Pts',(69.5049829210846,-1.16624389057502,
76.8561360003715));
#183624=CARTESIAN_POINT('Ctrl Pts',(72.2442227938533,-5.49870316824427,
76.4746767653586));
#183625=CARTESIAN_POINT('Ctrl Pts',(77.201853348837,-6.61409777385948,75.702055399319));
#183626=CARTESIAN_POINT('Ctrl Pts',(81.4858576528621,-3.85023340878249,
75.0482125162369));
#183627=CARTESIAN_POINT('Ctrl Pts',(82.6016717259066,1.16624389057504,74.9530070508935));
#183628=CARTESIAN_POINT('Ctrl Pts',(79.8971614886713,5.49870316824429,75.5314278365089));
#183629=CARTESIAN_POINT('Ctrl Pts',(74.9742605692209,6.61409777385949,76.5010107531509));
#183630=CARTESIAN_POINT('Ctrl Pts',(70.7249859007293,3.8502334087825,77.3518151868354));
#183631=CARTESIAN_POINT('Ctrl Pts',(69.6439014632181,-1.16624389057502,
77.6439822027812));
#183632=CARTESIAN_POINT('Ctrl Pts',(72.3831413359868,-5.49870316824427,
77.2625229677683));
#183633=CARTESIAN_POINT('Ctrl Pts',(77.3407718909705,-6.61409777385948,
76.4899016017287));
#183634=CARTESIAN_POINT('Ctrl Pts',(81.6247761949956,-3.85023340878248,
75.8360587186467));
#183635=CARTESIAN_POINT('Ctrl Pts',(82.7405902680401,1.16624389057503,75.7408532533033));
#183636=CARTESIAN_POINT('Ctrl Pts',(80.0360800308048,5.49870316824428,76.3192740389186));
#183637=CARTESIAN_POINT('Ctrl Pts',(75.1131791113545,6.6140977738595,77.2888569555607));
#183638=CARTESIAN_POINT('Ctrl Pts',(70.8639044428628,3.85023340878249,78.1396613892452));
#183639=CARTESIAN_POINT('Ctrl Pts',(69.7828200053516,-1.16624389057502,
78.431828405191));
#183640=CARTESIAN_POINT('Ctrl Pts',(72.5220598781203,-5.49870316824426,
78.0503691701781));
#183641=CARTESIAN_POINT('Ctrl Pts',(77.479690433104,-6.61409777385948,77.2777478041385));
#183642=CARTESIAN_POINT('Ctrl Pts',(81.7636947371291,-3.85023340878247,
76.6239049210564));
#183643=CARTESIAN_POINT('Ctrl Pts',(82.8795088101737,1.16624389057501,76.5286994557131));
#183644=CARTESIAN_POINT('Ctrl Pts',(80.1749985729384,5.49870316824428,77.1071202413284));
#183645=CARTESIAN_POINT('Ctrl Pts',(75.252097653488,6.61409777385949,78.0767031579704));
#183646=CARTESIAN_POINT('Ctrl Pts',(71.0028229849963,3.8502334087825,78.927507591655));
#183647=CARTESIAN_POINT('Ctrl Pts',(69.9217385474851,-1.16624389057503,
79.2196746076008));
#183648=CARTESIAN_POINT('Ctrl Pts',(72.6609784202538,-5.49870316824426,
78.8382153725879));
#183649=CARTESIAN_POINT('Ctrl Pts',(77.6186089752376,-6.61409777385948,
78.0655940065483));
#183650=CARTESIAN_POINT('Ctrl Pts',(81.9026132792626,-3.85023340878247,
77.4117511234662));
#183651=CARTESIAN_POINT('Ctrl Pts',(83.0184273523072,1.16624389057501,77.3165456581228));
#183652=CARTESIAN_POINT('Ctrl Pts',(80.3139171150719,5.49870316824428,77.8949664437382));
#183653=CARTESIAN_POINT('Ctrl Pts',(75.3910161956215,6.61409777385949,78.8645493603802));
#183654=CARTESIAN_POINT('Ctrl Pts',(71.1417415271298,3.8502334087825,79.7153537940648));
#183655=CARTESIAN_POINT('Ctrl Pts',(70.0606570896187,-1.16624389057503,
80.0075208100106));
#183656=CARTESIAN_POINT('Ctrl Pts',(72.7998969623873,-5.49870316824426,
79.6260615749977));
#183657=CARTESIAN_POINT('Ctrl Pts',(77.7575275173711,-6.61409777385948,
78.8534402089581));
#183658=CARTESIAN_POINT('Ctrl Pts',(82.0415318213962,-3.85023340878248,
78.199597325876));
#183659=CARTESIAN_POINT('Ctrl Pts',(83.1573458944407,1.16624389057501,78.1043918605326));
#183660=CARTESIAN_POINT('Ctrl Pts',(80.4528356572054,5.49870316824428,78.6828126461479));
#183661=CARTESIAN_POINT('Ctrl Pts',(75.529934737755,6.61409777385948,79.65239556279));
#183662=CARTESIAN_POINT('Ctrl Pts',(71.2806600692634,3.85023340878254,80.5031999964745));
#183663=CARTESIAN_POINT('Ctrl Pts',(70.1995756317522,-1.16624389057504,
80.7953670124203));
#183664=CARTESIAN_POINT('Ctrl Pts',(72.9388155045209,-5.49870316824426,
80.4139077774074));
#183665=CARTESIAN_POINT('Ctrl Pts',(77.8964460595046,-6.61409777385949,
79.6412864113678));
#183666=CARTESIAN_POINT('Ctrl Pts',(82.1804503635297,-3.85023340878247,
78.9874435282857));
#183667=CARTESIAN_POINT('Ctrl Pts',(83.2962644365742,1.166243890575,78.8922380629424));
#183668=CARTESIAN_POINT('Ctrl Pts',(80.5917541993389,5.49870316824431,79.4706588485577));
#183669=CARTESIAN_POINT('Ctrl Pts',(75.6688532798886,6.61409777385948,80.4402417651997));
#183670=CARTESIAN_POINT('Ctrl Pts',(71.4195786113969,3.85023340878254,81.2910461988843));
#183671=CARTESIAN_POINT('Ctrl Pts',(70.551115605666,-0.179632161764912,
81.5257514966757));
#183672=CARTESIAN_POINT('Ctrl Pts',(71.3088378859154,-2.31069653991403,
81.4398688991882));
#183673=CARTESIAN_POINT('Ctrl Pts',(71.6177826841475,-2.88208981923202,
81.3992703263852));
#183674=CARTESIAN_POINT('Ctrl Pts',(75.1229547057303,5.33099171449205,76.0413970676667));
#183675=CARTESIAN_POINT('Ctrl Pts',(73.7542956761902,5.08490089911617,76.3165761356943));
#183676=CARTESIAN_POINT('Ctrl Pts',(71.2285102044038,3.43952652893016,76.8296353693107));
#183677=CARTESIAN_POINT('Ctrl Pts',(70.2645980570925,-1.04183990292265,
77.1011417491029));
#183678=CARTESIAN_POINT('Ctrl Pts',(72.7134937630276,-4.91215295642792,
76.770878024394));
#183679=CARTESIAN_POINT('Ctrl Pts',(77.1441429869717,-5.90856770039853,
76.0911776853464));
#183680=CARTESIAN_POINT('Ctrl Pts',(80.9730221064147,-3.43952652893015,
75.517585651906));
#183681=CARTESIAN_POINT('Ctrl Pts',(81.9716638892593,1.04183990292267,75.4430408227163));
#183682=CARTESIAN_POINT('Ctrl Pts',(79.5574978188576,4.91215295642794,75.9702660980275));
#183683=CARTESIAN_POINT('Ctrl Pts',(75.161578230447,5.90856770039855,76.8469279876776));
#183684=CARTESIAN_POINT('Ctrl Pts',(71.3674287465373,3.43952652893017,77.6174815717205));
#183685=CARTESIAN_POINT('Ctrl Pts',(70.4035165992261,-1.04183990292265,
77.8889879515126));
#183686=CARTESIAN_POINT('Ctrl Pts',(72.8524123051612,-4.91215295642792,
77.5587242268038));
#183687=CARTESIAN_POINT('Ctrl Pts',(77.2830615291052,-5.90856770039853,
76.8790238877561));
#183688=CARTESIAN_POINT('Ctrl Pts',(81.1119406485482,-3.43952652893014,
76.3054318543158));
#183689=CARTESIAN_POINT('Ctrl Pts',(82.1105824313929,1.04183990292266,76.2308870251261));
#183690=CARTESIAN_POINT('Ctrl Pts',(79.6964163609912,4.91215295642793,76.7581123004373));
#183691=CARTESIAN_POINT('Ctrl Pts',(75.3004967725805,5.90856770039855,77.6347741900874));
#183692=CARTESIAN_POINT('Ctrl Pts',(71.5063472886708,3.43952652893016,78.4053277741302));
#183693=CARTESIAN_POINT('Ctrl Pts',(70.5424351413596,-1.04183990292265,
78.6768341539224));
#183694=CARTESIAN_POINT('Ctrl Pts',(72.9913308472947,-4.91215295642791,
78.3465704292136));
#183695=CARTESIAN_POINT('Ctrl Pts',(77.4219800712387,-5.90856770039854,
77.6668700901659));
#183696=CARTESIAN_POINT('Ctrl Pts',(81.2508591906818,-3.43952652893014,
77.0932780567255));
#183697=CARTESIAN_POINT('Ctrl Pts',(82.2495009735264,1.04183990292265,77.0187332275358));
#183698=CARTESIAN_POINT('Ctrl Pts',(79.8353349031247,4.91215295642793,77.5459585028471));
#183699=CARTESIAN_POINT('Ctrl Pts',(75.439415314714,5.90856770039855,78.4226203924972));
#183700=CARTESIAN_POINT('Ctrl Pts',(71.6452658308043,3.43952652893016,79.19317397654));
#183701=CARTESIAN_POINT('Ctrl Pts',(70.6813536834931,-1.04183990292266,
79.4646803563322));
#183702=CARTESIAN_POINT('Ctrl Pts',(73.1302493894282,-4.91215295642791,
79.1344166316234));
#183703=CARTESIAN_POINT('Ctrl Pts',(77.5608986133722,-5.90856770039854,
78.4547162925757));
#183704=CARTESIAN_POINT('Ctrl Pts',(81.3897777328153,-3.43952652893014,
77.8811242591353));
#183705=CARTESIAN_POINT('Ctrl Pts',(82.3884195156599,1.04183990292264,77.8065794299456));
#183706=CARTESIAN_POINT('Ctrl Pts',(79.9742534452582,4.91215295642793,78.3338047052569));
#183707=CARTESIAN_POINT('Ctrl Pts',(75.5783338568476,5.90856770039855,79.2104665949069));
#183708=CARTESIAN_POINT('Ctrl Pts',(71.7841843729379,3.43952652893017,79.9810201789498));
#183709=CARTESIAN_POINT('Ctrl Pts',(70.8202722256266,-1.04183990292266,
80.2525265587419));
#183710=CARTESIAN_POINT('Ctrl Pts',(73.2691679315617,-4.91215295642791,
79.9222628340331));
#183711=CARTESIAN_POINT('Ctrl Pts',(77.6998171555057,-5.90856770039854,
79.2425624949855));
#183712=CARTESIAN_POINT('Ctrl Pts',(81.5286962749488,-3.43952652893014,
78.6689704615451));
#183713=CARTESIAN_POINT('Ctrl Pts',(82.5273380577934,1.04183990292264,78.5944256323554));
#183714=CARTESIAN_POINT('Ctrl Pts',(80.1131719873917,4.91215295642793,79.1216509076666));
#183715=CARTESIAN_POINT('Ctrl Pts',(75.7172523989811,5.90856770039854,79.9983127973167));
#183716=CARTESIAN_POINT('Ctrl Pts',(71.9231029150714,3.4395265289302,80.7688663813595));
#183717=CARTESIAN_POINT('Ctrl Pts',(70.9591907677601,-1.04183990292267,
81.0403727611517));
#183718=CARTESIAN_POINT('Ctrl Pts',(73.4080864736952,-4.91215295642791,
80.7101090364429));
#183719=CARTESIAN_POINT('Ctrl Pts',(77.8387356976392,-5.90856770039855,
80.0304086973952));
#183720=CARTESIAN_POINT('Ctrl Pts',(81.6676148170823,-3.43952652893014,
79.4568166639549));
#183721=CARTESIAN_POINT('Ctrl Pts',(82.666256599927,1.04183990292264,79.3822718347651));
#183722=CARTESIAN_POINT('Ctrl Pts',(80.2520905295252,4.91215295642795,79.9094971100764));
#183723=CARTESIAN_POINT('Ctrl Pts',(75.8561709411146,5.90856770039853,80.7861589997265));
#183724=CARTESIAN_POINT('Ctrl Pts',(72.0620214572049,3.4395265289302,81.5567125837693));
#183725=CARTESIAN_POINT('Ctrl Pts',(71.2876859736217,-0.160470683265631,
81.7748206597788));
#183726=CARTESIAN_POINT('Ctrl Pts',(71.9654521044387,-2.06421305036014,
81.7030364887098));
#183727=CARTESIAN_POINT('Ctrl Pts',(72.2416946977908,-2.57465544021205,
81.6682041969559));
#183728=CARTESIAN_POINT('Origin',(79.2469596359123,7.105427357601E-15,94.016560397588));
#183729=CARTESIAN_POINT('',(72.7191598750949,4.47917030439226,95.1675876200822));
#183730=CARTESIAN_POINT('Origin',(72.7191598750949,4.47917030439226,95.1675876200822));
#183731=CARTESIAN_POINT('',(74.7096346164239,-3.98351688341825,97.8628930544244));
#183732=CARTESIAN_POINT('Ctrl Pts',(74.7096346161526,-3.98351688369326,
97.8628930549279));
#183733=CARTESIAN_POINT('Ctrl Pts',(74.7227886043145,-4.12739717889162,
97.7913931478345));
#183734=CARTESIAN_POINT('Ctrl Pts',(74.7353899189023,-4.27253790874392,
97.7154740533153));
#183735=CARTESIAN_POINT('Ctrl Pts',(74.7474888928844,-4.41924001704132,
97.6351268963102));
#183736=CARTESIAN_POINT('Ctrl Pts',(74.7597998396111,-4.56851233076134,
97.5533720656115));
#183737=CARTESIAN_POINT('Ctrl Pts',(74.7715915811878,-4.71940100604202,
97.4670324976694));
#183738=CARTESIAN_POINT('Ctrl Pts',(74.7829106449292,-4.87217012296937,
97.3760999884628));
#183739=CARTESIAN_POINT('Ctrl Pts',(74.7843368471221,-4.89141903388181,
97.3646424910054));
#183740=CARTESIAN_POINT('Ctrl Pts',(74.785755526609,-4.91069773354052,97.353112079253));
#183741=CARTESIAN_POINT('Ctrl Pts',(74.7871667585286,-4.93000669486555,
97.3415087399564));
#183742=CARTESIAN_POINT('',(73.2401044080956,4.47917030439226,98.1220108791188));
#183743=CARTESIAN_POINT('Origin',(79.2469596359123,7.105427357601E-15,94.016560397588));
#183744=CARTESIAN_POINT('',(85.7747593967297,-4.47917030439225,92.8655331750938));
#183745=CARTESIAN_POINT('Origin',(85.7747593967297,-4.47917030439225,92.8655331750938));
#183746=CARTESIAN_POINT('',(85.862867185943,-1.98656284024888,95.8962772303022));
#183747=CARTESIAN_POINT('',(86.2957039297304,-4.47917030439225,95.8199564341304));
#183748=CARTESIAN_POINT('Ctrl Pts',(85.9403993280472,-2.93305265169037,
95.3748929158375));
#183749=CARTESIAN_POINT('Ctrl Pts',(85.9045302932766,-2.44228015705023,
95.6698129624946));
#183750=CARTESIAN_POINT('Ctrl Pts',(85.8628671861297,-1.98656284058723,
95.8962772310178));
#183751=CARTESIAN_POINT('Origin',(76.8158851485756,7.14546725904962E-15,
80.229251855417));
#183752=CARTESIAN_POINT('Origin',(76.1212924379081,7.15881389286582E-15,
76.2900208433682));
#183753=CARTESIAN_POINT('Origin',(76.9027092374091,7.105427357601E-15,80.7216557319231));
#183754=CARTESIAN_POINT('Origin',(79.6810800800795,7.105427357601E-15,96.4785797801185));
#183755=CARTESIAN_POINT('Origin',(79.767904168913,7.105427357601E-15,96.9709836566246));
#183756=CARTESIAN_POINT('Origin',(79.767904168913,7.105427357601E-15,96.9709836566246));
#221642=UNCERTAINTY_MEASURE_WITH_UNIT(LENGTH_MEASURE(0.01),#221663,
'DISTANCE_ACCURACY_VALUE',
'Maximum model space distance between geometric entities at asserted c
onnectivities');
#221647=UNCERTAINTY_MEASURE_WITH_UNIT(LENGTH_MEASURE(0.01),#221663,
'DISTANCE_ACCURACY_VALUE',
'Maximum model space distance between geometric entities at asserted c
onnectivities');
#221657=(
GEOMETRIC_REPRESENTATION_CONTEXT(3)
GLOBAL_UNCERTAINTY_ASSIGNED_CONTEXT((#221642))
GLOBAL_UNIT_ASSIGNED_CONTEXT((#221663,#221665,#221666))
REPRESENTATION_CONTEXT('','3D')
);
#221662=(
GEOMETRIC_REPRESENTATION_CONTEXT(3)
GLOBAL_UNCERTAINTY_ASSIGNED_CONTEXT((#221647))
GLOBAL_UNIT_ASSIGNED_CONTEXT((#221663,#221665,#221666))
REPRESENTATION_CONTEXT('','3D')
);
#221663=(
LENGTH_UNIT()
NAMED_UNIT(*)
SI_UNIT(.MILLI.,.METRE.)
);
#221665=(
NAMED_UNIT(*)
PLANE_ANGLE_UNIT()
SI_UNIT($,.RADIAN.)
);
#221666=(
NAMED_UNIT(*)
SI_UNIT($,.STERADIAN.)
SOLID_ANGLE_UNIT()
);
#221676=SHAPE_DEFINITION_REPRESENTATION(#221690,#221717);
#221690=PRODUCT_DEFINITION_SHAPE('',$,#221732);
#221717=SHAPE_REPRESENTATION('',(#80848),#221657);
#221722=PRODUCT_DEFINITION_CONTEXT('part definition',#221766,'design');
#221732=PRODUCT_DEFINITION('2026-10-05-23-02-42-253','Diverter',#221746,
#221722);
#221746=PRODUCT_DEFINITION_FORMATION('',$,#221777);
#221766=APPLICATION_CONTEXT(
'Core Data for Automotive Mechanical Design Process');
#221767=PRODUCT_CONTEXT('part definition',#221766,'mechanical');
#221777=PRODUCT('2026-10-05-23-02-42-253','Diverter',$,(#221767));
#221783=PRESENTATION_STYLE_ASSIGNMENT((#221785));
#221785=SURFACE_STYLE_USAGE(.BOTH.,#221787);
#221787=SURFACE_SIDE_STYLE('',(#221789));
#221789=SURFACE_STYLE_FILL_AREA(#221791);
#221791=FILL_AREA_STYLE('Opaque(202,209,238)',(#221793));
#221793=FILL_AREA_STYLE_COLOUR('Opaque(202,209,238)',#221795);
#221795=COLOUR_RGB('Opaque(202,209,238)', 0.09019608, 0.27058824, 0.51372549);
ENDSEC;
END-ISO-10303-21;
